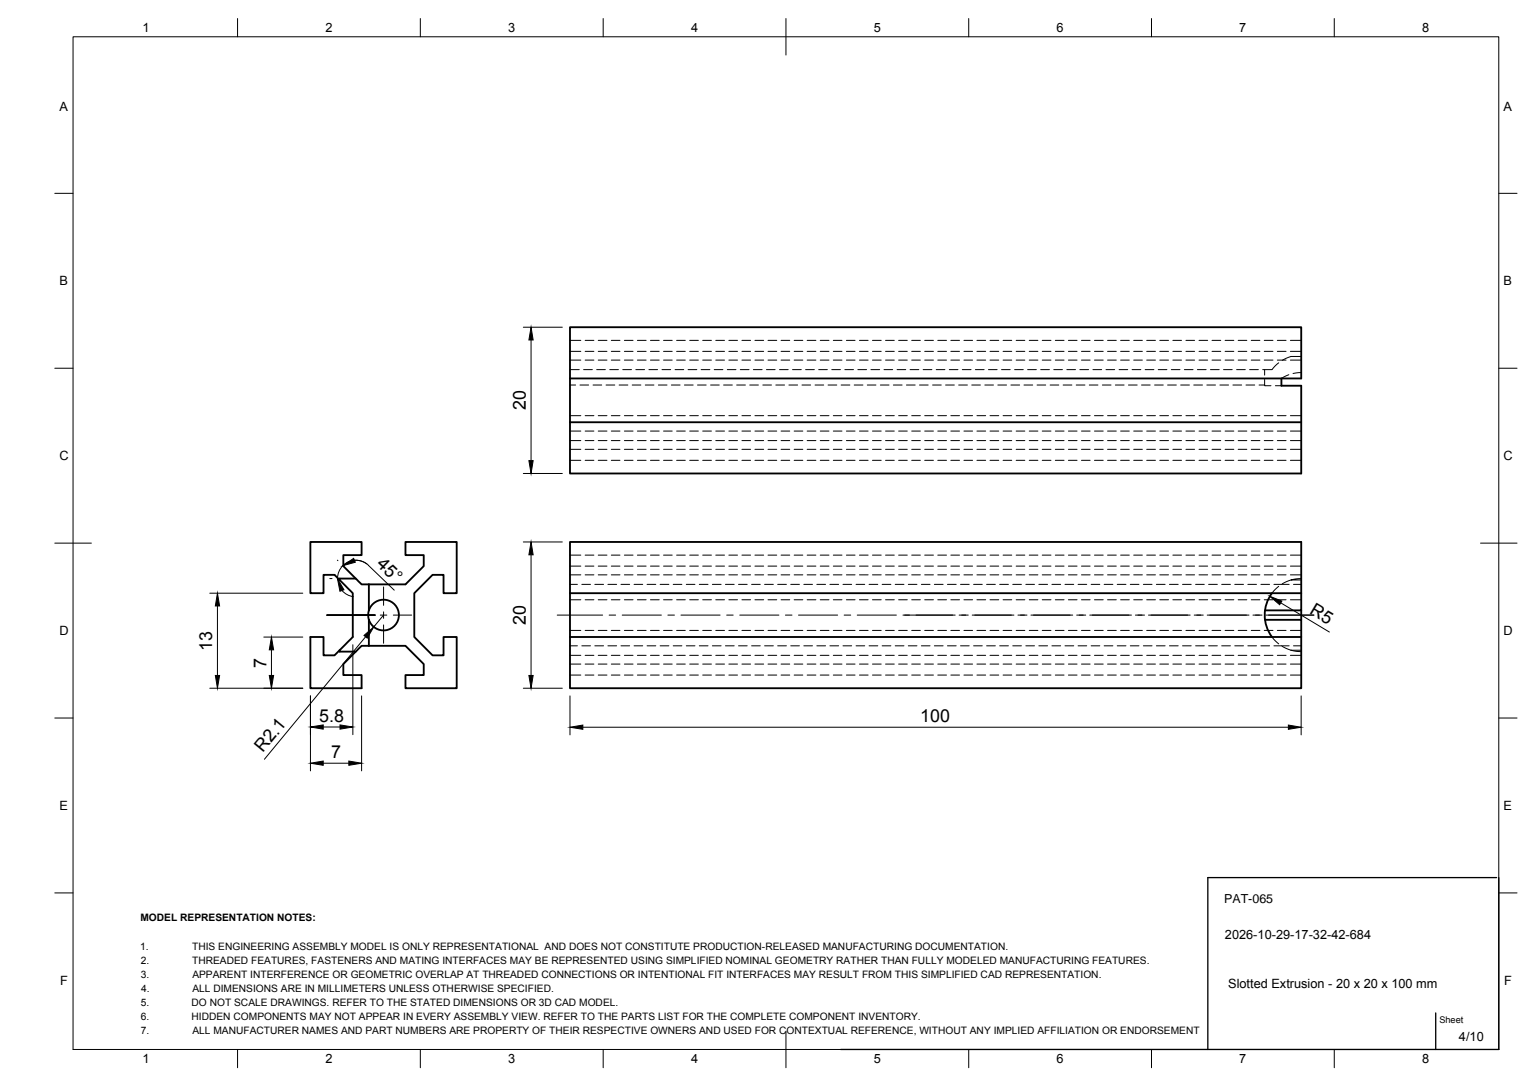
ISO-10303-21;
HEADER;
/* Generated by software containing ST-Developer
 * from STEP Tools, Inc. (www.steptools.com) 
 */

FILE_DESCRIPTION(
/* description */ ('PAT-065'),
/* implementation_level */ '2;1');

FILE_NAME(
/* name */ 'Slotted Extrusion - 20 x 20 x 100 mm.step',
/* time_stamp */ '2026-10-28T22:09:22-07:00',
/* author */ (''),
/* organization */ (''),
/* preprocessor_version */ 'ST-DEVELOPER v20.2',
/* originating_system */ 'Autodesk Translation Framework v15.17.0.0',
/* authorisation */ '');

FILE_SCHEMA (('AUTOMOTIVE_DESIGN { 1 0 10303 214 3 1 1 }'));
ENDSEC;

DATA;
#10=MECHANICAL_DESIGN_GEOMETRIC_PRESENTATION_REPRESENTATION('',(#159),#5502);
#128=B_SPLINE_CURVE_WITH_KNOTS('',3,(#4608,#4609,#4610,#4611,#4612,#4613),
 .UNSPECIFIED.,.F.,.F.,(4,2,4),(0.899292285450093,0.96236755734344,1.02544282923679),
 .UNSPECIFIED.);
#129=ELLIPSE('',#3350,0.707106781186548,0.5);
#130=ELLIPSE('',#3352,0.707106781186547,0.5);
#131=ELLIPSE('',#3354,0.707106781186548,0.5);
#132=ELLIPSE('',#3355,0.707106781186548,0.5);
#139=SHAPE_REPRESENTATION_RELATIONSHIP('SRR','None',#5556,#149);
#149=ADVANCED_BREP_SHAPE_REPRESENTATION('',(#169),#5492);
#159=STYLED_ITEM('',(#5708),#169);
#169=MANIFOLD_SOLID_BREP('Body1',#3206);
#183=FACE_BOUND('',#579,.T.);
#207=PLANE('',#3345);
#208=PLANE('',#3347);
#209=PLANE('',#3357);
#210=PLANE('',#3358);
#211=PLANE('',#3359);
#212=PLANE('',#3360);
#213=PLANE('',#3361);
#214=PLANE('',#3362);
#215=PLANE('',#3363);
#216=PLANE('',#3364);
#217=PLANE('',#3367);
#218=PLANE('',#3368);
#219=PLANE('',#3369);
#220=PLANE('',#3370);
#221=PLANE('',#3371);
#222=PLANE('',#3372);
#223=PLANE('',#3373);
#224=PLANE('',#3374);
#225=PLANE('',#3375);
#226=PLANE('',#3376);
#227=PLANE('',#3377);
#228=PLANE('',#3378);
#229=PLANE('',#3379);
#230=PLANE('',#3380);
#231=PLANE('',#3381);
#232=PLANE('',#3382);
#233=PLANE('',#3383);
#234=PLANE('',#3384);
#235=PLANE('',#3385);
#236=PLANE('',#3386);
#237=PLANE('',#3387);
#238=PLANE('',#3388);
#239=PLANE('',#3389);
#240=PLANE('',#3390);
#241=PLANE('',#3391);
#242=PLANE('',#3392);
#243=PLANE('',#3393);
#244=PLANE('',#3394);
#245=PLANE('',#3395);
#246=PLANE('',#3396);
#247=PLANE('',#3397);
#248=PLANE('',#3398);
#249=PLANE('',#3401);
#250=PLANE('',#3402);
#251=PLANE('',#3403);
#252=PLANE('',#3404);
#253=PLANE('',#3405);
#254=PLANE('',#3406);
#255=PLANE('',#3407);
#256=PLANE('',#3408);
#257=PLANE('',#3409);
#258=PLANE('',#3410);
#346=FACE_OUTER_BOUND('',#526,.T.);
#347=FACE_OUTER_BOUND('',#527,.T.);
#348=FACE_OUTER_BOUND('',#528,.T.);
#349=FACE_OUTER_BOUND('',#529,.T.);
#350=FACE_OUTER_BOUND('',#530,.T.);
#351=FACE_OUTER_BOUND('',#531,.T.);
#352=FACE_OUTER_BOUND('',#532,.T.);
#353=FACE_OUTER_BOUND('',#533,.T.);
#354=FACE_OUTER_BOUND('',#534,.T.);
#355=FACE_OUTER_BOUND('',#535,.T.);
#356=FACE_OUTER_BOUND('',#536,.T.);
#357=FACE_OUTER_BOUND('',#537,.T.);
#358=FACE_OUTER_BOUND('',#538,.T.);
#359=FACE_OUTER_BOUND('',#539,.T.);
#360=FACE_OUTER_BOUND('',#540,.T.);
#361=FACE_OUTER_BOUND('',#541,.T.);
#362=FACE_OUTER_BOUND('',#542,.T.);
#363=FACE_OUTER_BOUND('',#543,.T.);
#364=FACE_OUTER_BOUND('',#544,.T.);
#365=FACE_OUTER_BOUND('',#545,.T.);
#366=FACE_OUTER_BOUND('',#546,.T.);
#367=FACE_OUTER_BOUND('',#547,.T.);
#368=FACE_OUTER_BOUND('',#548,.T.);
#369=FACE_OUTER_BOUND('',#549,.T.);
#370=FACE_OUTER_BOUND('',#550,.T.);
#371=FACE_OUTER_BOUND('',#551,.T.);
#372=FACE_OUTER_BOUND('',#552,.T.);
#373=FACE_OUTER_BOUND('',#553,.T.);
#374=FACE_OUTER_BOUND('',#554,.T.);
#375=FACE_OUTER_BOUND('',#555,.T.);
#376=FACE_OUTER_BOUND('',#556,.T.);
#377=FACE_OUTER_BOUND('',#557,.T.);
#378=FACE_OUTER_BOUND('',#558,.T.);
#379=FACE_OUTER_BOUND('',#559,.T.);
#380=FACE_OUTER_BOUND('',#560,.T.);
#381=FACE_OUTER_BOUND('',#561,.T.);
#382=FACE_OUTER_BOUND('',#562,.T.);
#383=FACE_OUTER_BOUND('',#563,.T.);
#384=FACE_OUTER_BOUND('',#564,.T.);
#385=FACE_OUTER_BOUND('',#565,.T.);
#386=FACE_OUTER_BOUND('',#566,.T.);
#387=FACE_OUTER_BOUND('',#567,.T.);
#388=FACE_OUTER_BOUND('',#568,.T.);
#389=FACE_OUTER_BOUND('',#569,.T.);
#390=FACE_OUTER_BOUND('',#570,.T.);
#391=FACE_OUTER_BOUND('',#571,.T.);
#392=FACE_OUTER_BOUND('',#572,.T.);
#393=FACE_OUTER_BOUND('',#573,.T.);
#394=FACE_OUTER_BOUND('',#574,.T.);
#395=FACE_OUTER_BOUND('',#575,.T.);
#396=FACE_OUTER_BOUND('',#576,.T.);
#397=FACE_OUTER_BOUND('',#577,.T.);
#398=FACE_OUTER_BOUND('',#578,.T.);
#399=FACE_OUTER_BOUND('',#580,.T.);
#526=EDGE_LOOP('',(#2194,#2195,#2196));
#527=EDGE_LOOP('',(#2197,#2198,#2199,#2200));
#528=EDGE_LOOP('',(#2201,#2202,#2203,#2204,#2205,#2206,#2207,#2208,#2209,
#2210,#2211,#2212,#2213,#2214));
#529=EDGE_LOOP('',(#2215,#2216,#2217));
#530=EDGE_LOOP('',(#2218,#2219,#2220,#2221));
#531=EDGE_LOOP('',(#2222,#2223,#2224,#2225));
#532=EDGE_LOOP('',(#2226,#2227,#2228,#2229,#2230,#2231));
#533=EDGE_LOOP('',(#2232,#2233,#2234,#2235,#2236));
#534=EDGE_LOOP('',(#2237,#2238,#2239,#2240,#2241,#2242));
#535=EDGE_LOOP('',(#2243,#2244,#2245,#2246,#2247,#2248,#2249,#2250,#2251,
#2252,#2253,#2254));
#536=EDGE_LOOP('',(#2255,#2256,#2257,#2258,#2259,#2260,#2261,#2262,#2263,
#2264,#2265,#2266,#2267,#2268,#2269,#2270,#2271,#2272,#2273,#2274,#2275,
#2276,#2277,#2278,#2279,#2280,#2281));
#537=EDGE_LOOP('',(#2282,#2283,#2284,#2285));
#538=EDGE_LOOP('',(#2286,#2287,#2288,#2289));
#539=EDGE_LOOP('',(#2290,#2291,#2292,#2293));
#540=EDGE_LOOP('',(#2294,#2295,#2296,#2297,#2298,#2299));
#541=EDGE_LOOP('',(#2300,#2301,#2302,#2303));
#542=EDGE_LOOP('',(#2304,#2305,#2306,#2307));
#543=EDGE_LOOP('',(#2308,#2309,#2310,#2311));
#544=EDGE_LOOP('',(#2312,#2313,#2314,#2315));
#545=EDGE_LOOP('',(#2316,#2317,#2318,#2319));
#546=EDGE_LOOP('',(#2320,#2321,#2322,#2323));
#547=EDGE_LOOP('',(#2324,#2325,#2326,#2327));
#548=EDGE_LOOP('',(#2328,#2329,#2330,#2331,#2332,#2333));
#549=EDGE_LOOP('',(#2334,#2335,#2336,#2337,#2338));
#550=EDGE_LOOP('',(#2339,#2340,#2341,#2342));
#551=EDGE_LOOP('',(#2343,#2344,#2345,#2346));
#552=EDGE_LOOP('',(#2347,#2348,#2349,#2350));
#553=EDGE_LOOP('',(#2351,#2352,#2353,#2354));
#554=EDGE_LOOP('',(#2355,#2356,#2357,#2358));
#555=EDGE_LOOP('',(#2359,#2360,#2361,#2362));
#556=EDGE_LOOP('',(#2363,#2364,#2365,#2366));
#557=EDGE_LOOP('',(#2367,#2368,#2369,#2370));
#558=EDGE_LOOP('',(#2371,#2372,#2373,#2374));
#559=EDGE_LOOP('',(#2375,#2376,#2377,#2378));
#560=EDGE_LOOP('',(#2379,#2380,#2381,#2382));
#561=EDGE_LOOP('',(#2383,#2384,#2385,#2386));
#562=EDGE_LOOP('',(#2387,#2388,#2389,#2390));
#563=EDGE_LOOP('',(#2391,#2392,#2393,#2394));
#564=EDGE_LOOP('',(#2395,#2396,#2397,#2398));
#565=EDGE_LOOP('',(#2399,#2400,#2401,#2402));
#566=EDGE_LOOP('',(#2403,#2404,#2405,#2406));
#567=EDGE_LOOP('',(#2407,#2408,#2409,#2410));
#568=EDGE_LOOP('',(#2411,#2412,#2413,#2414));
#569=EDGE_LOOP('',(#2415,#2416,#2417,#2418,#2419,#2420,#2421,#2422));
#570=EDGE_LOOP('',(#2423,#2424,#2425,#2426));
#571=EDGE_LOOP('',(#2427,#2428,#2429,#2430));
#572=EDGE_LOOP('',(#2431,#2432,#2433,#2434));
#573=EDGE_LOOP('',(#2435,#2436,#2437,#2438));
#574=EDGE_LOOP('',(#2439,#2440,#2441,#2442));
#575=EDGE_LOOP('',(#2443,#2444,#2445,#2446));
#576=EDGE_LOOP('',(#2447,#2448,#2449,#2450));
#577=EDGE_LOOP('',(#2451,#2452,#2453,#2454));
#578=EDGE_LOOP('',(#2455,#2456,#2457,#2458,#2459,#2460,#2461,#2462,#2463,
#2464,#2465,#2466,#2467,#2468,#2469,#2470,#2471,#2472,#2473,#2474,#2475,
#2476,#2477,#2478,#2479,#2480,#2481,#2482,#2483,#2484,#2485,#2486,#2487,
#2488,#2489,#2490,#2491,#2492,#2493,#2494,#2495,#2496,#2497,#2498));
#579=EDGE_LOOP('',(#2499));
#580=EDGE_LOOP('',(#2500,#2501,#2502,#2503,#2504,#2505,#2506,#2507,#2508,
#2509,#2510,#2511));
#724=LINE('',#4581,#1055);
#725=LINE('',#4584,#1056);
#726=LINE('',#4588,#1057);
#727=LINE('',#4592,#1058);
#728=LINE('',#4593,#1059);
#729=LINE('',#4601,#1060);
#730=LINE('',#4605,#1061);
#731=LINE('',#4615,#1062);
#732=LINE('',#4618,#1063);
#733=LINE('',#4624,#1064);
#734=LINE('',#4625,#1065);
#735=LINE('',#4628,#1066);
#736=LINE('',#4630,#1067);
#737=LINE('',#4631,#1068);
#738=LINE('',#4634,#1069);
#739=LINE('',#4636,#1070);
#740=LINE('',#4637,#1071);
#741=LINE('',#4640,#1072);
#742=LINE('',#4642,#1073);
#743=LINE('',#4643,#1074);
#744=LINE('',#4646,#1075);
#745=LINE('',#4648,#1076);
#746=LINE('',#4650,#1077);
#747=LINE('',#4651,#1078);
#748=LINE('',#4654,#1079);
#749=LINE('',#4656,#1080);
#750=LINE('',#4657,#1081);
#751=LINE('',#4660,#1082);
#752=LINE('',#4662,#1083);
#753=LINE('',#4664,#1084);
#754=LINE('',#4666,#1085);
#755=LINE('',#4668,#1086);
#756=LINE('',#4670,#1087);
#757=LINE('',#4672,#1088);
#758=LINE('',#4673,#1089);
#759=LINE('',#4676,#1090);
#760=LINE('',#4678,#1091);
#761=LINE('',#4680,#1092);
#762=LINE('',#4682,#1093);
#763=LINE('',#4684,#1094);
#764=LINE('',#4686,#1095);
#765=LINE('',#4688,#1096);
#766=LINE('',#4690,#1097);
#767=LINE('',#4692,#1098);
#768=LINE('',#4694,#1099);
#769=LINE('',#4696,#1100);
#770=LINE('',#4698,#1101);
#771=LINE('',#4700,#1102);
#772=LINE('',#4702,#1103);
#773=LINE('',#4704,#1104);
#774=LINE('',#4706,#1105);
#775=LINE('',#4708,#1106);
#776=LINE('',#4710,#1107);
#777=LINE('',#4712,#1108);
#778=LINE('',#4714,#1109);
#779=LINE('',#4716,#1110);
#780=LINE('',#4717,#1111);
#781=LINE('',#4724,#1112);
#782=LINE('',#4726,#1113);
#783=LINE('',#4728,#1114);
#784=LINE('',#4729,#1115);
#785=LINE('',#4732,#1116);
#786=LINE('',#4734,#1117);
#787=LINE('',#4735,#1118);
#788=LINE('',#4738,#1119);
#789=LINE('',#4740,#1120);
#790=LINE('',#4741,#1121);
#791=LINE('',#4743,#1122);
#792=LINE('',#4744,#1123);
#793=LINE('',#4747,#1124);
#794=LINE('',#4748,#1125);
#795=LINE('',#4751,#1126);
#796=LINE('',#4752,#1127);
#797=LINE('',#4755,#1128);
#798=LINE('',#4756,#1129);
#799=LINE('',#4759,#1130);
#800=LINE('',#4761,#1131);
#801=LINE('',#4762,#1132);
#802=LINE('',#4765,#1133);
#803=LINE('',#4766,#1134);
#804=LINE('',#4769,#1135);
#805=LINE('',#4770,#1136);
#806=LINE('',#4773,#1137);
#807=LINE('',#4774,#1138);
#808=LINE('',#4777,#1139);
#809=LINE('',#4778,#1140);
#810=LINE('',#4781,#1141);
#811=LINE('',#4783,#1142);
#812=LINE('',#4784,#1143);
#813=LINE('',#4787,#1144);
#814=LINE('',#4789,#1145);
#815=LINE('',#4790,#1146);
#816=LINE('',#4793,#1147);
#817=LINE('',#4795,#1148);
#818=LINE('',#4796,#1149);
#819=LINE('',#4799,#1150);
#820=LINE('',#4801,#1151);
#821=LINE('',#4802,#1152);
#822=LINE('',#4805,#1153);
#823=LINE('',#4807,#1154);
#824=LINE('',#4808,#1155);
#825=LINE('',#4811,#1156);
#826=LINE('',#4812,#1157);
#827=LINE('',#4815,#1158);
#828=LINE('',#4816,#1159);
#829=LINE('',#4819,#1160);
#830=LINE('',#4820,#1161);
#831=LINE('',#4823,#1162);
#832=LINE('',#4824,#1163);
#833=LINE('',#4827,#1164);
#834=LINE('',#4828,#1165);
#835=LINE('',#4831,#1166);
#836=LINE('',#4832,#1167);
#837=LINE('',#4835,#1168);
#838=LINE('',#4836,#1169);
#839=LINE('',#4839,#1170);
#840=LINE('',#4840,#1171);
#841=LINE('',#4843,#1172);
#842=LINE('',#4845,#1173);
#843=LINE('',#4846,#1174);
#844=LINE('',#4849,#1175);
#845=LINE('',#4850,#1176);
#846=LINE('',#4852,#1177);
#847=LINE('',#4855,#1178);
#848=LINE('',#4856,#1179);
#849=LINE('',#4859,#1180);
#850=LINE('',#4860,#1181);
#851=LINE('',#4863,#1182);
#852=LINE('',#4864,#1183);
#853=LINE('',#4867,#1184);
#854=LINE('',#4868,#1185);
#855=LINE('',#4871,#1186);
#856=LINE('',#4875,#1187);
#857=LINE('',#4876,#1188);
#858=LINE('',#4879,#1189);
#859=LINE('',#4881,#1190);
#860=LINE('',#4882,#1191);
#861=LINE('',#4884,#1192);
#862=LINE('',#4885,#1193);
#863=LINE('',#4888,#1194);
#864=LINE('',#4889,#1195);
#865=LINE('',#4891,#1196);
#866=LINE('',#4894,#1197);
#867=LINE('',#4895,#1198);
#868=LINE('',#4897,#1199);
#869=LINE('',#4899,#1200);
#1055=VECTOR('',#3671,1.);
#1056=VECTOR('',#3674,1.);
#1057=VECTOR('',#3677,1.);
#1058=VECTOR('',#3680,1.);
#1059=VECTOR('',#3681,1.);
#1060=VECTOR('',#3688,1.);
#1061=VECTOR('',#3691,1.);
#1062=VECTOR('',#3694,1.);
#1063=VECTOR('',#3697,1.);
#1064=VECTOR('',#3704,1.);
#1065=VECTOR('',#3705,1.);
#1066=VECTOR('',#3708,1.);
#1067=VECTOR('',#3709,1.);
#1068=VECTOR('',#3710,1.);
#1069=VECTOR('',#3713,1.);
#1070=VECTOR('',#3714,1.);
#1071=VECTOR('',#3715,1.);
#1072=VECTOR('',#3718,1.);
#1073=VECTOR('',#3719,1.);
#1074=VECTOR('',#3720,1.);
#1075=VECTOR('',#3723,1.);
#1076=VECTOR('',#3724,1.);
#1077=VECTOR('',#3725,1.);
#1078=VECTOR('',#3726,1.);
#1079=VECTOR('',#3729,1.);
#1080=VECTOR('',#3730,1.);
#1081=VECTOR('',#3731,1.);
#1082=VECTOR('',#3734,1.);
#1083=VECTOR('',#3735,1.);
#1084=VECTOR('',#3736,1.);
#1085=VECTOR('',#3737,1.);
#1086=VECTOR('',#3738,1.);
#1087=VECTOR('',#3739,1.);
#1088=VECTOR('',#3740,1.);
#1089=VECTOR('',#3741,1.);
#1090=VECTOR('',#3744,1.);
#1091=VECTOR('',#3745,1.);
#1092=VECTOR('',#3746,1.);
#1093=VECTOR('',#3747,1.);
#1094=VECTOR('',#3748,1.);
#1095=VECTOR('',#3749,1.);
#1096=VECTOR('',#3750,1.);
#1097=VECTOR('',#3751,1.);
#1098=VECTOR('',#3752,1.);
#1099=VECTOR('',#3753,1.);
#1100=VECTOR('',#3754,1.);
#1101=VECTOR('',#3755,1.);
#1102=VECTOR('',#3756,1.);
#1103=VECTOR('',#3757,1.);
#1104=VECTOR('',#3758,1.);
#1105=VECTOR('',#3759,1.);
#1106=VECTOR('',#3760,1.);
#1107=VECTOR('',#3761,1.);
#1108=VECTOR('',#3762,1.);
#1109=VECTOR('',#3763,1.);
#1110=VECTOR('',#3764,1.);
#1111=VECTOR('',#3765,1.);
#1112=VECTOR('',#3772,1.);
#1113=VECTOR('',#3773,1.);
#1114=VECTOR('',#3774,1.);
#1115=VECTOR('',#3775,1.);
#1116=VECTOR('',#3778,1.);
#1117=VECTOR('',#3779,1.);
#1118=VECTOR('',#3780,1.);
#1119=VECTOR('',#3783,1.);
#1120=VECTOR('',#3784,1.);
#1121=VECTOR('',#3785,1.);
#1122=VECTOR('',#3788,1.);
#1123=VECTOR('',#3789,1.);
#1124=VECTOR('',#3792,1.);
#1125=VECTOR('',#3793,1.);
#1126=VECTOR('',#3796,1.);
#1127=VECTOR('',#3797,1.);
#1128=VECTOR('',#3800,1.);
#1129=VECTOR('',#3801,1.);
#1130=VECTOR('',#3804,1.);
#1131=VECTOR('',#3805,1.);
#1132=VECTOR('',#3806,1.);
#1133=VECTOR('',#3809,1.);
#1134=VECTOR('',#3810,1.);
#1135=VECTOR('',#3813,1.);
#1136=VECTOR('',#3814,1.);
#1137=VECTOR('',#3817,1.);
#1138=VECTOR('',#3818,1.);
#1139=VECTOR('',#3821,1.);
#1140=VECTOR('',#3822,1.);
#1141=VECTOR('',#3825,1.);
#1142=VECTOR('',#3826,1.);
#1143=VECTOR('',#3827,1.);
#1144=VECTOR('',#3830,1.);
#1145=VECTOR('',#3831,1.);
#1146=VECTOR('',#3832,1.);
#1147=VECTOR('',#3835,1.);
#1148=VECTOR('',#3836,1.);
#1149=VECTOR('',#3837,1.);
#1150=VECTOR('',#3840,1.);
#1151=VECTOR('',#3841,1.);
#1152=VECTOR('',#3842,1.);
#1153=VECTOR('',#3845,1.);
#1154=VECTOR('',#3846,1.);
#1155=VECTOR('',#3847,1.);
#1156=VECTOR('',#3850,1.);
#1157=VECTOR('',#3851,1.);
#1158=VECTOR('',#3854,1.);
#1159=VECTOR('',#3855,1.);
#1160=VECTOR('',#3858,1.);
#1161=VECTOR('',#3859,1.);
#1162=VECTOR('',#3862,1.);
#1163=VECTOR('',#3863,1.);
#1164=VECTOR('',#3866,1.);
#1165=VECTOR('',#3867,1.);
#1166=VECTOR('',#3870,1.);
#1167=VECTOR('',#3871,1.);
#1168=VECTOR('',#3874,1.);
#1169=VECTOR('',#3875,1.);
#1170=VECTOR('',#3878,1.);
#1171=VECTOR('',#3879,1.);
#1172=VECTOR('',#3882,1.);
#1173=VECTOR('',#3883,1.);
#1174=VECTOR('',#3884,1.);
#1175=VECTOR('',#3887,1.);
#1176=VECTOR('',#3888,1.);
#1177=VECTOR('',#3891,1.);
#1178=VECTOR('',#3894,1.);
#1179=VECTOR('',#3895,1.);
#1180=VECTOR('',#3898,1.);
#1181=VECTOR('',#3899,1.);
#1182=VECTOR('',#3902,1.);
#1183=VECTOR('',#3903,1.);
#1184=VECTOR('',#3906,1.);
#1185=VECTOR('',#3907,1.);
#1186=VECTOR('',#3910,0.21);
#1187=VECTOR('',#3915,1.);
#1188=VECTOR('',#3916,1.);
#1189=VECTOR('',#3919,1.);
#1190=VECTOR('',#3920,1.);
#1191=VECTOR('',#3921,1.);
#1192=VECTOR('',#3924,1.);
#1193=VECTOR('',#3925,1.);
#1194=VECTOR('',#3928,1.);
#1195=VECTOR('',#3929,1.);
#1196=VECTOR('',#3932,1.);
#1197=VECTOR('',#3935,1.);
#1198=VECTOR('',#3936,1.);
#1199=VECTOR('',#3939,1.);
#1200=VECTOR('',#3942,1.);
#1377=CIRCLE('',#3346,0.5);
#1378=CIRCLE('',#3348,0.5);
#1379=CIRCLE('',#3351,0.5);
#1380=CIRCLE('',#3353,0.5);
#1381=CIRCLE('',#3356,0.5);
#1382=CIRCLE('',#3365,0.21);
#1383=CIRCLE('',#3366,0.21);
#1384=CIRCLE('',#3400,0.21);
#1458=VERTEX_POINT('',#4579);
#1459=VERTEX_POINT('',#4580);
#1460=VERTEX_POINT('',#4582);
#1461=VERTEX_POINT('',#4586);
#1462=VERTEX_POINT('',#4587);
#1463=VERTEX_POINT('',#4589);
#1464=VERTEX_POINT('',#4591);
#1465=VERTEX_POINT('',#4595);
#1466=VERTEX_POINT('',#4596);
#1467=VERTEX_POINT('',#4598);
#1468=VERTEX_POINT('',#4600);
#1469=VERTEX_POINT('',#4602);
#1470=VERTEX_POINT('',#4604);
#1471=VERTEX_POINT('',#4606);
#1472=VERTEX_POINT('',#4614);
#1473=VERTEX_POINT('',#4616);
#1474=VERTEX_POINT('',#4619);
#1475=VERTEX_POINT('',#4623);
#1476=VERTEX_POINT('',#4627);
#1477=VERTEX_POINT('',#4629);
#1478=VERTEX_POINT('',#4633);
#1479=VERTEX_POINT('',#4635);
#1480=VERTEX_POINT('',#4639);
#1481=VERTEX_POINT('',#4641);
#1482=VERTEX_POINT('',#4645);
#1483=VERTEX_POINT('',#4647);
#1484=VERTEX_POINT('',#4649);
#1485=VERTEX_POINT('',#4653);
#1486=VERTEX_POINT('',#4655);
#1487=VERTEX_POINT('',#4659);
#1488=VERTEX_POINT('',#4661);
#1489=VERTEX_POINT('',#4663);
#1490=VERTEX_POINT('',#4665);
#1491=VERTEX_POINT('',#4667);
#1492=VERTEX_POINT('',#4669);
#1493=VERTEX_POINT('',#4671);
#1494=VERTEX_POINT('',#4675);
#1495=VERTEX_POINT('',#4677);
#1496=VERTEX_POINT('',#4679);
#1497=VERTEX_POINT('',#4681);
#1498=VERTEX_POINT('',#4683);
#1499=VERTEX_POINT('',#4685);
#1500=VERTEX_POINT('',#4687);
#1501=VERTEX_POINT('',#4689);
#1502=VERTEX_POINT('',#4691);
#1503=VERTEX_POINT('',#4693);
#1504=VERTEX_POINT('',#4695);
#1505=VERTEX_POINT('',#4697);
#1506=VERTEX_POINT('',#4699);
#1507=VERTEX_POINT('',#4701);
#1508=VERTEX_POINT('',#4703);
#1509=VERTEX_POINT('',#4705);
#1510=VERTEX_POINT('',#4707);
#1511=VERTEX_POINT('',#4709);
#1512=VERTEX_POINT('',#4711);
#1513=VERTEX_POINT('',#4713);
#1514=VERTEX_POINT('',#4715);
#1515=VERTEX_POINT('',#4718);
#1516=VERTEX_POINT('',#4722);
#1517=VERTEX_POINT('',#4723);
#1518=VERTEX_POINT('',#4725);
#1519=VERTEX_POINT('',#4727);
#1520=VERTEX_POINT('',#4731);
#1521=VERTEX_POINT('',#4733);
#1522=VERTEX_POINT('',#4737);
#1523=VERTEX_POINT('',#4739);
#1524=VERTEX_POINT('',#4746);
#1525=VERTEX_POINT('',#4750);
#1526=VERTEX_POINT('',#4754);
#1527=VERTEX_POINT('',#4758);
#1528=VERTEX_POINT('',#4760);
#1529=VERTEX_POINT('',#4764);
#1530=VERTEX_POINT('',#4768);
#1531=VERTEX_POINT('',#4772);
#1532=VERTEX_POINT('',#4776);
#1533=VERTEX_POINT('',#4780);
#1534=VERTEX_POINT('',#4782);
#1535=VERTEX_POINT('',#4786);
#1536=VERTEX_POINT('',#4788);
#1537=VERTEX_POINT('',#4792);
#1538=VERTEX_POINT('',#4794);
#1539=VERTEX_POINT('',#4798);
#1540=VERTEX_POINT('',#4800);
#1541=VERTEX_POINT('',#4804);
#1542=VERTEX_POINT('',#4806);
#1543=VERTEX_POINT('',#4810);
#1544=VERTEX_POINT('',#4814);
#1545=VERTEX_POINT('',#4818);
#1546=VERTEX_POINT('',#4822);
#1547=VERTEX_POINT('',#4826);
#1548=VERTEX_POINT('',#4830);
#1549=VERTEX_POINT('',#4834);
#1550=VERTEX_POINT('',#4838);
#1551=VERTEX_POINT('',#4842);
#1552=VERTEX_POINT('',#4844);
#1553=VERTEX_POINT('',#4848);
#1554=VERTEX_POINT('',#4854);
#1555=VERTEX_POINT('',#4858);
#1556=VERTEX_POINT('',#4862);
#1557=VERTEX_POINT('',#4866);
#1558=VERTEX_POINT('',#4870);
#1559=VERTEX_POINT('',#4874);
#1560=VERTEX_POINT('',#4878);
#1561=VERTEX_POINT('',#4880);
#1562=VERTEX_POINT('',#4887);
#1563=VERTEX_POINT('',#4893);
#1747=EDGE_CURVE('',#1458,#1459,#724,.T.);
#1748=EDGE_CURVE('',#1460,#1458,#1377,.T.);
#1749=EDGE_CURVE('',#1459,#1460,#725,.T.);
#1750=EDGE_CURVE('',#1461,#1462,#726,.T.);
#1751=EDGE_CURVE('',#1461,#1463,#1378,.T.);
#1752=EDGE_CURVE('',#1464,#1463,#727,.T.);
#1753=EDGE_CURVE('',#1462,#1464,#728,.T.);
#1754=EDGE_CURVE('',#1465,#1466,#129,.T.);
#1755=EDGE_CURVE('',#1465,#1467,#1379,.T.);
#1756=EDGE_CURVE('',#1468,#1467,#729,.T.);
#1757=EDGE_CURVE('',#1469,#1468,#130,.T.);
#1758=EDGE_CURVE('',#1470,#1469,#730,.T.);
#1759=EDGE_CURVE('',#1471,#1470,#1380,.T.);
#1760=EDGE_CURVE('',#1463,#1471,#128,.T.);
#1761=EDGE_CURVE('',#1472,#1461,#731,.T.);
#1762=EDGE_CURVE('',#1473,#1472,#131,.T.);
#1763=EDGE_CURVE('',#1460,#1473,#732,.T.);
#1764=EDGE_CURVE('',#1474,#1458,#132,.T.);
#1765=EDGE_CURVE('',#1466,#1474,#1381,.T.);
#1766=EDGE_CURVE('',#1475,#1465,#733,.T.);
#1767=EDGE_CURVE('',#1467,#1475,#734,.T.);
#1768=EDGE_CURVE('',#1476,#1470,#735,.T.);
#1769=EDGE_CURVE('',#1477,#1476,#736,.T.);
#1770=EDGE_CURVE('',#1471,#1477,#737,.T.);
#1771=EDGE_CURVE('',#1474,#1478,#738,.T.);
#1772=EDGE_CURVE('',#1479,#1478,#739,.T.);
#1773=EDGE_CURVE('',#1466,#1479,#740,.T.);
#1774=EDGE_CURVE('',#1480,#1459,#741,.T.);
#1775=EDGE_CURVE('',#1480,#1481,#742,.T.);
#1776=EDGE_CURVE('',#1478,#1481,#743,.T.);
#1777=EDGE_CURVE('',#1472,#1482,#744,.T.);
#1778=EDGE_CURVE('',#1483,#1482,#745,.T.);
#1779=EDGE_CURVE('',#1484,#1483,#746,.T.);
#1780=EDGE_CURVE('',#1473,#1484,#747,.T.);
#1781=EDGE_CURVE('',#1485,#1462,#748,.T.);
#1782=EDGE_CURVE('',#1485,#1486,#749,.T.);
#1783=EDGE_CURVE('',#1482,#1486,#750,.T.);
#1784=EDGE_CURVE('',#1484,#1487,#751,.T.);
#1785=EDGE_CURVE('',#1487,#1488,#752,.T.);
#1786=EDGE_CURVE('',#1488,#1489,#753,.T.);
#1787=EDGE_CURVE('',#1490,#1489,#754,.T.);
#1788=EDGE_CURVE('',#1491,#1490,#755,.T.);
#1789=EDGE_CURVE('',#1491,#1492,#756,.T.);
#1790=EDGE_CURVE('',#1492,#1493,#757,.T.);
#1791=EDGE_CURVE('',#1493,#1480,#758,.T.);
#1792=EDGE_CURVE('',#1476,#1494,#759,.T.);
#1793=EDGE_CURVE('',#1494,#1495,#760,.T.);
#1794=EDGE_CURVE('',#1495,#1496,#761,.T.);
#1795=EDGE_CURVE('',#1496,#1497,#762,.T.);
#1796=EDGE_CURVE('',#1497,#1498,#763,.T.);
#1797=EDGE_CURVE('',#1499,#1498,#764,.T.);
#1798=EDGE_CURVE('',#1500,#1499,#765,.T.);
#1799=EDGE_CURVE('',#1500,#1501,#766,.T.);
#1800=EDGE_CURVE('',#1501,#1502,#767,.T.);
#1801=EDGE_CURVE('',#1502,#1503,#768,.T.);
#1802=EDGE_CURVE('',#1503,#1504,#769,.T.);
#1803=EDGE_CURVE('',#1504,#1505,#770,.T.);
#1804=EDGE_CURVE('',#1505,#1506,#771,.T.);
#1805=EDGE_CURVE('',#1506,#1507,#772,.T.);
#1806=EDGE_CURVE('',#1507,#1508,#773,.T.);
#1807=EDGE_CURVE('',#1508,#1509,#774,.T.);
#1808=EDGE_CURVE('',#1510,#1509,#775,.T.);
#1809=EDGE_CURVE('',#1511,#1510,#776,.T.);
#1810=EDGE_CURVE('',#1511,#1512,#777,.T.);
#1811=EDGE_CURVE('',#1512,#1513,#778,.T.);
#1812=EDGE_CURVE('',#1513,#1514,#779,.T.);
#1813=EDGE_CURVE('',#1514,#1485,#780,.T.);
#1814=EDGE_CURVE('',#1464,#1515,#1382,.T.);
#1815=EDGE_CURVE('',#1515,#1477,#1383,.T.);
#1816=EDGE_CURVE('',#1516,#1517,#781,.T.);
#1817=EDGE_CURVE('',#1516,#1518,#782,.T.);
#1818=EDGE_CURVE('',#1519,#1518,#783,.T.);
#1819=EDGE_CURVE('',#1517,#1519,#784,.T.);
#1820=EDGE_CURVE('',#1520,#1516,#785,.T.);
#1821=EDGE_CURVE('',#1520,#1521,#786,.T.);
#1822=EDGE_CURVE('',#1518,#1521,#787,.T.);
#1823=EDGE_CURVE('',#1522,#1520,#788,.T.);
#1824=EDGE_CURVE('',#1522,#1523,#789,.T.);
#1825=EDGE_CURVE('',#1521,#1523,#790,.T.);
#1826=EDGE_CURVE('',#1523,#1479,#791,.T.);
#1827=EDGE_CURVE('',#1475,#1522,#792,.T.);
#1828=EDGE_CURVE('',#1493,#1524,#793,.T.);
#1829=EDGE_CURVE('',#1481,#1524,#794,.T.);
#1830=EDGE_CURVE('',#1492,#1525,#795,.T.);
#1831=EDGE_CURVE('',#1524,#1525,#796,.T.);
#1832=EDGE_CURVE('',#1526,#1491,#797,.T.);
#1833=EDGE_CURVE('',#1525,#1526,#798,.T.);
#1834=EDGE_CURVE('',#1497,#1527,#799,.T.);
#1835=EDGE_CURVE('',#1528,#1527,#800,.T.);
#1836=EDGE_CURVE('',#1498,#1528,#801,.T.);
#1837=EDGE_CURVE('',#1496,#1529,#802,.T.);
#1838=EDGE_CURVE('',#1527,#1529,#803,.T.);
#1839=EDGE_CURVE('',#1495,#1530,#804,.T.);
#1840=EDGE_CURVE('',#1529,#1530,#805,.T.);
#1841=EDGE_CURVE('',#1494,#1531,#806,.T.);
#1842=EDGE_CURVE('',#1530,#1531,#807,.T.);
#1843=EDGE_CURVE('',#1469,#1532,#808,.T.);
#1844=EDGE_CURVE('',#1531,#1532,#809,.T.);
#1845=EDGE_CURVE('',#1533,#1468,#810,.T.);
#1846=EDGE_CURVE('',#1533,#1534,#811,.T.);
#1847=EDGE_CURVE('',#1532,#1534,#812,.T.);
#1848=EDGE_CURVE('',#1535,#1533,#813,.T.);
#1849=EDGE_CURVE('',#1535,#1536,#814,.T.);
#1850=EDGE_CURVE('',#1534,#1536,#815,.T.);
#1851=EDGE_CURVE('',#1537,#1535,#816,.T.);
#1852=EDGE_CURVE('',#1537,#1538,#817,.T.);
#1853=EDGE_CURVE('',#1536,#1538,#818,.T.);
#1854=EDGE_CURVE('',#1539,#1537,#819,.T.);
#1855=EDGE_CURVE('',#1540,#1539,#820,.T.);
#1856=EDGE_CURVE('',#1538,#1540,#821,.T.);
#1857=EDGE_CURVE('',#1508,#1541,#822,.T.);
#1858=EDGE_CURVE('',#1542,#1541,#823,.T.);
#1859=EDGE_CURVE('',#1509,#1542,#824,.T.);
#1860=EDGE_CURVE('',#1507,#1543,#825,.T.);
#1861=EDGE_CURVE('',#1541,#1543,#826,.T.);
#1862=EDGE_CURVE('',#1506,#1544,#827,.T.);
#1863=EDGE_CURVE('',#1543,#1544,#828,.T.);
#1864=EDGE_CURVE('',#1505,#1545,#829,.T.);
#1865=EDGE_CURVE('',#1544,#1545,#830,.T.);
#1866=EDGE_CURVE('',#1504,#1546,#831,.T.);
#1867=EDGE_CURVE('',#1545,#1546,#832,.T.);
#1868=EDGE_CURVE('',#1503,#1547,#833,.T.);
#1869=EDGE_CURVE('',#1546,#1547,#834,.T.);
#1870=EDGE_CURVE('',#1502,#1548,#835,.T.);
#1871=EDGE_CURVE('',#1547,#1548,#836,.T.);
#1872=EDGE_CURVE('',#1501,#1549,#837,.T.);
#1873=EDGE_CURVE('',#1548,#1549,#838,.T.);
#1874=EDGE_CURVE('',#1550,#1500,#839,.T.);
#1875=EDGE_CURVE('',#1549,#1550,#840,.T.);
#1876=EDGE_CURVE('',#1488,#1551,#841,.T.);
#1877=EDGE_CURVE('',#1552,#1551,#842,.T.);
#1878=EDGE_CURVE('',#1489,#1552,#843,.T.);
#1879=EDGE_CURVE('',#1487,#1553,#844,.T.);
#1880=EDGE_CURVE('',#1551,#1553,#845,.T.);
#1881=EDGE_CURVE('',#1553,#1483,#846,.T.);
#1882=EDGE_CURVE('',#1514,#1554,#847,.T.);
#1883=EDGE_CURVE('',#1486,#1554,#848,.T.);
#1884=EDGE_CURVE('',#1513,#1555,#849,.T.);
#1885=EDGE_CURVE('',#1554,#1555,#850,.T.);
#1886=EDGE_CURVE('',#1512,#1556,#851,.T.);
#1887=EDGE_CURVE('',#1555,#1556,#852,.T.);
#1888=EDGE_CURVE('',#1557,#1511,#853,.T.);
#1889=EDGE_CURVE('',#1556,#1557,#854,.T.);
#1890=EDGE_CURVE('',#1515,#1558,#855,.T.);
#1891=EDGE_CURVE('',#1558,#1558,#1384,.T.);
#1892=EDGE_CURVE('',#1490,#1559,#856,.T.);
#1893=EDGE_CURVE('',#1526,#1559,#857,.T.);
#1894=EDGE_CURVE('',#1560,#1519,#858,.T.);
#1895=EDGE_CURVE('',#1561,#1560,#859,.T.);
#1896=EDGE_CURVE('',#1561,#1517,#860,.T.);
#1897=EDGE_CURVE('',#1539,#1561,#861,.T.);
#1898=EDGE_CURVE('',#1540,#1560,#862,.T.);
#1899=EDGE_CURVE('',#1562,#1528,#863,.T.);
#1900=EDGE_CURVE('',#1499,#1562,#864,.T.);
#1901=EDGE_CURVE('',#1550,#1562,#865,.T.);
#1902=EDGE_CURVE('',#1563,#1542,#866,.T.);
#1903=EDGE_CURVE('',#1510,#1563,#867,.T.);
#1904=EDGE_CURVE('',#1557,#1563,#868,.T.);
#1905=EDGE_CURVE('',#1559,#1552,#869,.T.);
#2194=ORIENTED_EDGE('',*,*,#1747,.F.);
#2195=ORIENTED_EDGE('',*,*,#1748,.F.);
#2196=ORIENTED_EDGE('',*,*,#1749,.F.);
#2197=ORIENTED_EDGE('',*,*,#1750,.F.);
#2198=ORIENTED_EDGE('',*,*,#1751,.T.);
#2199=ORIENTED_EDGE('',*,*,#1752,.F.);
#2200=ORIENTED_EDGE('',*,*,#1753,.F.);
#2201=ORIENTED_EDGE('',*,*,#1754,.F.);
#2202=ORIENTED_EDGE('',*,*,#1755,.T.);
#2203=ORIENTED_EDGE('',*,*,#1756,.F.);
#2204=ORIENTED_EDGE('',*,*,#1757,.F.);
#2205=ORIENTED_EDGE('',*,*,#1758,.F.);
#2206=ORIENTED_EDGE('',*,*,#1759,.F.);
#2207=ORIENTED_EDGE('',*,*,#1760,.F.);
#2208=ORIENTED_EDGE('',*,*,#1751,.F.);
#2209=ORIENTED_EDGE('',*,*,#1761,.F.);
#2210=ORIENTED_EDGE('',*,*,#1762,.F.);
#2211=ORIENTED_EDGE('',*,*,#1763,.F.);
#2212=ORIENTED_EDGE('',*,*,#1748,.T.);
#2213=ORIENTED_EDGE('',*,*,#1764,.F.);
#2214=ORIENTED_EDGE('',*,*,#1765,.F.);
#2215=ORIENTED_EDGE('',*,*,#1766,.F.);
#2216=ORIENTED_EDGE('',*,*,#1767,.F.);
#2217=ORIENTED_EDGE('',*,*,#1755,.F.);
#2218=ORIENTED_EDGE('',*,*,#1768,.F.);
#2219=ORIENTED_EDGE('',*,*,#1769,.F.);
#2220=ORIENTED_EDGE('',*,*,#1770,.F.);
#2221=ORIENTED_EDGE('',*,*,#1759,.T.);
#2222=ORIENTED_EDGE('',*,*,#1765,.T.);
#2223=ORIENTED_EDGE('',*,*,#1771,.T.);
#2224=ORIENTED_EDGE('',*,*,#1772,.F.);
#2225=ORIENTED_EDGE('',*,*,#1773,.F.);
#2226=ORIENTED_EDGE('',*,*,#1764,.T.);
#2227=ORIENTED_EDGE('',*,*,#1747,.T.);
#2228=ORIENTED_EDGE('',*,*,#1774,.F.);
#2229=ORIENTED_EDGE('',*,*,#1775,.T.);
#2230=ORIENTED_EDGE('',*,*,#1776,.F.);
#2231=ORIENTED_EDGE('',*,*,#1771,.F.);
#2232=ORIENTED_EDGE('',*,*,#1762,.T.);
#2233=ORIENTED_EDGE('',*,*,#1777,.T.);
#2234=ORIENTED_EDGE('',*,*,#1778,.F.);
#2235=ORIENTED_EDGE('',*,*,#1779,.F.);
#2236=ORIENTED_EDGE('',*,*,#1780,.F.);
#2237=ORIENTED_EDGE('',*,*,#1761,.T.);
#2238=ORIENTED_EDGE('',*,*,#1750,.T.);
#2239=ORIENTED_EDGE('',*,*,#1781,.F.);
#2240=ORIENTED_EDGE('',*,*,#1782,.T.);
#2241=ORIENTED_EDGE('',*,*,#1783,.F.);
#2242=ORIENTED_EDGE('',*,*,#1777,.F.);
#2243=ORIENTED_EDGE('',*,*,#1749,.T.);
#2244=ORIENTED_EDGE('',*,*,#1763,.T.);
#2245=ORIENTED_EDGE('',*,*,#1780,.T.);
#2246=ORIENTED_EDGE('',*,*,#1784,.T.);
#2247=ORIENTED_EDGE('',*,*,#1785,.T.);
#2248=ORIENTED_EDGE('',*,*,#1786,.T.);
#2249=ORIENTED_EDGE('',*,*,#1787,.F.);
#2250=ORIENTED_EDGE('',*,*,#1788,.F.);
#2251=ORIENTED_EDGE('',*,*,#1789,.T.);
#2252=ORIENTED_EDGE('',*,*,#1790,.T.);
#2253=ORIENTED_EDGE('',*,*,#1791,.T.);
#2254=ORIENTED_EDGE('',*,*,#1774,.T.);
#2255=ORIENTED_EDGE('',*,*,#1769,.T.);
#2256=ORIENTED_EDGE('',*,*,#1792,.T.);
#2257=ORIENTED_EDGE('',*,*,#1793,.T.);
#2258=ORIENTED_EDGE('',*,*,#1794,.T.);
#2259=ORIENTED_EDGE('',*,*,#1795,.T.);
#2260=ORIENTED_EDGE('',*,*,#1796,.T.);
#2261=ORIENTED_EDGE('',*,*,#1797,.F.);
#2262=ORIENTED_EDGE('',*,*,#1798,.F.);
#2263=ORIENTED_EDGE('',*,*,#1799,.T.);
#2264=ORIENTED_EDGE('',*,*,#1800,.T.);
#2265=ORIENTED_EDGE('',*,*,#1801,.T.);
#2266=ORIENTED_EDGE('',*,*,#1802,.T.);
#2267=ORIENTED_EDGE('',*,*,#1803,.T.);
#2268=ORIENTED_EDGE('',*,*,#1804,.T.);
#2269=ORIENTED_EDGE('',*,*,#1805,.T.);
#2270=ORIENTED_EDGE('',*,*,#1806,.T.);
#2271=ORIENTED_EDGE('',*,*,#1807,.T.);
#2272=ORIENTED_EDGE('',*,*,#1808,.F.);
#2273=ORIENTED_EDGE('',*,*,#1809,.F.);
#2274=ORIENTED_EDGE('',*,*,#1810,.T.);
#2275=ORIENTED_EDGE('',*,*,#1811,.T.);
#2276=ORIENTED_EDGE('',*,*,#1812,.T.);
#2277=ORIENTED_EDGE('',*,*,#1813,.T.);
#2278=ORIENTED_EDGE('',*,*,#1781,.T.);
#2279=ORIENTED_EDGE('',*,*,#1753,.T.);
#2280=ORIENTED_EDGE('',*,*,#1814,.T.);
#2281=ORIENTED_EDGE('',*,*,#1815,.T.);
#2282=ORIENTED_EDGE('',*,*,#1816,.F.);
#2283=ORIENTED_EDGE('',*,*,#1817,.T.);
#2284=ORIENTED_EDGE('',*,*,#1818,.F.);
#2285=ORIENTED_EDGE('',*,*,#1819,.F.);
#2286=ORIENTED_EDGE('',*,*,#1820,.F.);
#2287=ORIENTED_EDGE('',*,*,#1821,.T.);
#2288=ORIENTED_EDGE('',*,*,#1822,.F.);
#2289=ORIENTED_EDGE('',*,*,#1817,.F.);
#2290=ORIENTED_EDGE('',*,*,#1823,.F.);
#2291=ORIENTED_EDGE('',*,*,#1824,.T.);
#2292=ORIENTED_EDGE('',*,*,#1825,.F.);
#2293=ORIENTED_EDGE('',*,*,#1821,.F.);
#2294=ORIENTED_EDGE('',*,*,#1754,.T.);
#2295=ORIENTED_EDGE('',*,*,#1773,.T.);
#2296=ORIENTED_EDGE('',*,*,#1826,.F.);
#2297=ORIENTED_EDGE('',*,*,#1824,.F.);
#2298=ORIENTED_EDGE('',*,*,#1827,.F.);
#2299=ORIENTED_EDGE('',*,*,#1766,.T.);
#2300=ORIENTED_EDGE('',*,*,#1791,.F.);
#2301=ORIENTED_EDGE('',*,*,#1828,.T.);
#2302=ORIENTED_EDGE('',*,*,#1829,.F.);
#2303=ORIENTED_EDGE('',*,*,#1775,.F.);
#2304=ORIENTED_EDGE('',*,*,#1790,.F.);
#2305=ORIENTED_EDGE('',*,*,#1830,.T.);
#2306=ORIENTED_EDGE('',*,*,#1831,.F.);
#2307=ORIENTED_EDGE('',*,*,#1828,.F.);
#2308=ORIENTED_EDGE('',*,*,#1789,.F.);
#2309=ORIENTED_EDGE('',*,*,#1832,.F.);
#2310=ORIENTED_EDGE('',*,*,#1833,.F.);
#2311=ORIENTED_EDGE('',*,*,#1830,.F.);
#2312=ORIENTED_EDGE('',*,*,#1796,.F.);
#2313=ORIENTED_EDGE('',*,*,#1834,.T.);
#2314=ORIENTED_EDGE('',*,*,#1835,.F.);
#2315=ORIENTED_EDGE('',*,*,#1836,.F.);
#2316=ORIENTED_EDGE('',*,*,#1795,.F.);
#2317=ORIENTED_EDGE('',*,*,#1837,.T.);
#2318=ORIENTED_EDGE('',*,*,#1838,.F.);
#2319=ORIENTED_EDGE('',*,*,#1834,.F.);
#2320=ORIENTED_EDGE('',*,*,#1794,.F.);
#2321=ORIENTED_EDGE('',*,*,#1839,.T.);
#2322=ORIENTED_EDGE('',*,*,#1840,.F.);
#2323=ORIENTED_EDGE('',*,*,#1837,.F.);
#2324=ORIENTED_EDGE('',*,*,#1793,.F.);
#2325=ORIENTED_EDGE('',*,*,#1841,.T.);
#2326=ORIENTED_EDGE('',*,*,#1842,.F.);
#2327=ORIENTED_EDGE('',*,*,#1839,.F.);
#2328=ORIENTED_EDGE('',*,*,#1758,.T.);
#2329=ORIENTED_EDGE('',*,*,#1843,.T.);
#2330=ORIENTED_EDGE('',*,*,#1844,.F.);
#2331=ORIENTED_EDGE('',*,*,#1841,.F.);
#2332=ORIENTED_EDGE('',*,*,#1792,.F.);
#2333=ORIENTED_EDGE('',*,*,#1768,.T.);
#2334=ORIENTED_EDGE('',*,*,#1757,.T.);
#2335=ORIENTED_EDGE('',*,*,#1845,.F.);
#2336=ORIENTED_EDGE('',*,*,#1846,.T.);
#2337=ORIENTED_EDGE('',*,*,#1847,.F.);
#2338=ORIENTED_EDGE('',*,*,#1843,.F.);
#2339=ORIENTED_EDGE('',*,*,#1848,.F.);
#2340=ORIENTED_EDGE('',*,*,#1849,.T.);
#2341=ORIENTED_EDGE('',*,*,#1850,.F.);
#2342=ORIENTED_EDGE('',*,*,#1846,.F.);
#2343=ORIENTED_EDGE('',*,*,#1851,.F.);
#2344=ORIENTED_EDGE('',*,*,#1852,.T.);
#2345=ORIENTED_EDGE('',*,*,#1853,.F.);
#2346=ORIENTED_EDGE('',*,*,#1849,.F.);
#2347=ORIENTED_EDGE('',*,*,#1854,.F.);
#2348=ORIENTED_EDGE('',*,*,#1855,.F.);
#2349=ORIENTED_EDGE('',*,*,#1856,.F.);
#2350=ORIENTED_EDGE('',*,*,#1852,.F.);
#2351=ORIENTED_EDGE('',*,*,#1807,.F.);
#2352=ORIENTED_EDGE('',*,*,#1857,.T.);
#2353=ORIENTED_EDGE('',*,*,#1858,.F.);
#2354=ORIENTED_EDGE('',*,*,#1859,.F.);
#2355=ORIENTED_EDGE('',*,*,#1806,.F.);
#2356=ORIENTED_EDGE('',*,*,#1860,.T.);
#2357=ORIENTED_EDGE('',*,*,#1861,.F.);
#2358=ORIENTED_EDGE('',*,*,#1857,.F.);
#2359=ORIENTED_EDGE('',*,*,#1805,.F.);
#2360=ORIENTED_EDGE('',*,*,#1862,.T.);
#2361=ORIENTED_EDGE('',*,*,#1863,.F.);
#2362=ORIENTED_EDGE('',*,*,#1860,.F.);
#2363=ORIENTED_EDGE('',*,*,#1804,.F.);
#2364=ORIENTED_EDGE('',*,*,#1864,.T.);
#2365=ORIENTED_EDGE('',*,*,#1865,.F.);
#2366=ORIENTED_EDGE('',*,*,#1862,.F.);
#2367=ORIENTED_EDGE('',*,*,#1803,.F.);
#2368=ORIENTED_EDGE('',*,*,#1866,.T.);
#2369=ORIENTED_EDGE('',*,*,#1867,.F.);
#2370=ORIENTED_EDGE('',*,*,#1864,.F.);
#2371=ORIENTED_EDGE('',*,*,#1802,.F.);
#2372=ORIENTED_EDGE('',*,*,#1868,.T.);
#2373=ORIENTED_EDGE('',*,*,#1869,.F.);
#2374=ORIENTED_EDGE('',*,*,#1866,.F.);
#2375=ORIENTED_EDGE('',*,*,#1801,.F.);
#2376=ORIENTED_EDGE('',*,*,#1870,.T.);
#2377=ORIENTED_EDGE('',*,*,#1871,.F.);
#2378=ORIENTED_EDGE('',*,*,#1868,.F.);
#2379=ORIENTED_EDGE('',*,*,#1800,.F.);
#2380=ORIENTED_EDGE('',*,*,#1872,.T.);
#2381=ORIENTED_EDGE('',*,*,#1873,.F.);
#2382=ORIENTED_EDGE('',*,*,#1870,.F.);
#2383=ORIENTED_EDGE('',*,*,#1799,.F.);
#2384=ORIENTED_EDGE('',*,*,#1874,.F.);
#2385=ORIENTED_EDGE('',*,*,#1875,.F.);
#2386=ORIENTED_EDGE('',*,*,#1872,.F.);
#2387=ORIENTED_EDGE('',*,*,#1786,.F.);
#2388=ORIENTED_EDGE('',*,*,#1876,.T.);
#2389=ORIENTED_EDGE('',*,*,#1877,.F.);
#2390=ORIENTED_EDGE('',*,*,#1878,.F.);
#2391=ORIENTED_EDGE('',*,*,#1785,.F.);
#2392=ORIENTED_EDGE('',*,*,#1879,.T.);
#2393=ORIENTED_EDGE('',*,*,#1880,.F.);
#2394=ORIENTED_EDGE('',*,*,#1876,.F.);
#2395=ORIENTED_EDGE('',*,*,#1784,.F.);
#2396=ORIENTED_EDGE('',*,*,#1779,.T.);
#2397=ORIENTED_EDGE('',*,*,#1881,.F.);
#2398=ORIENTED_EDGE('',*,*,#1879,.F.);
#2399=ORIENTED_EDGE('',*,*,#1813,.F.);
#2400=ORIENTED_EDGE('',*,*,#1882,.T.);
#2401=ORIENTED_EDGE('',*,*,#1883,.F.);
#2402=ORIENTED_EDGE('',*,*,#1782,.F.);
#2403=ORIENTED_EDGE('',*,*,#1812,.F.);
#2404=ORIENTED_EDGE('',*,*,#1884,.T.);
#2405=ORIENTED_EDGE('',*,*,#1885,.F.);
#2406=ORIENTED_EDGE('',*,*,#1882,.F.);
#2407=ORIENTED_EDGE('',*,*,#1811,.F.);
#2408=ORIENTED_EDGE('',*,*,#1886,.T.);
#2409=ORIENTED_EDGE('',*,*,#1887,.F.);
#2410=ORIENTED_EDGE('',*,*,#1884,.F.);
#2411=ORIENTED_EDGE('',*,*,#1810,.F.);
#2412=ORIENTED_EDGE('',*,*,#1888,.F.);
#2413=ORIENTED_EDGE('',*,*,#1889,.F.);
#2414=ORIENTED_EDGE('',*,*,#1886,.F.);
#2415=ORIENTED_EDGE('',*,*,#1770,.T.);
#2416=ORIENTED_EDGE('',*,*,#1815,.F.);
#2417=ORIENTED_EDGE('',*,*,#1890,.T.);
#2418=ORIENTED_EDGE('',*,*,#1891,.F.);
#2419=ORIENTED_EDGE('',*,*,#1890,.F.);
#2420=ORIENTED_EDGE('',*,*,#1814,.F.);
#2421=ORIENTED_EDGE('',*,*,#1752,.T.);
#2422=ORIENTED_EDGE('',*,*,#1760,.T.);
#2423=ORIENTED_EDGE('',*,*,#1832,.T.);
#2424=ORIENTED_EDGE('',*,*,#1788,.T.);
#2425=ORIENTED_EDGE('',*,*,#1892,.T.);
#2426=ORIENTED_EDGE('',*,*,#1893,.F.);
#2427=ORIENTED_EDGE('',*,*,#1819,.T.);
#2428=ORIENTED_EDGE('',*,*,#1894,.F.);
#2429=ORIENTED_EDGE('',*,*,#1895,.F.);
#2430=ORIENTED_EDGE('',*,*,#1896,.T.);
#2431=ORIENTED_EDGE('',*,*,#1855,.T.);
#2432=ORIENTED_EDGE('',*,*,#1897,.T.);
#2433=ORIENTED_EDGE('',*,*,#1895,.T.);
#2434=ORIENTED_EDGE('',*,*,#1898,.F.);
#2435=ORIENTED_EDGE('',*,*,#1836,.T.);
#2436=ORIENTED_EDGE('',*,*,#1899,.F.);
#2437=ORIENTED_EDGE('',*,*,#1900,.F.);
#2438=ORIENTED_EDGE('',*,*,#1797,.T.);
#2439=ORIENTED_EDGE('',*,*,#1874,.T.);
#2440=ORIENTED_EDGE('',*,*,#1798,.T.);
#2441=ORIENTED_EDGE('',*,*,#1900,.T.);
#2442=ORIENTED_EDGE('',*,*,#1901,.F.);
#2443=ORIENTED_EDGE('',*,*,#1859,.T.);
#2444=ORIENTED_EDGE('',*,*,#1902,.F.);
#2445=ORIENTED_EDGE('',*,*,#1903,.F.);
#2446=ORIENTED_EDGE('',*,*,#1808,.T.);
#2447=ORIENTED_EDGE('',*,*,#1888,.T.);
#2448=ORIENTED_EDGE('',*,*,#1809,.T.);
#2449=ORIENTED_EDGE('',*,*,#1903,.T.);
#2450=ORIENTED_EDGE('',*,*,#1904,.F.);
#2451=ORIENTED_EDGE('',*,*,#1878,.T.);
#2452=ORIENTED_EDGE('',*,*,#1905,.F.);
#2453=ORIENTED_EDGE('',*,*,#1892,.F.);
#2454=ORIENTED_EDGE('',*,*,#1787,.T.);
#2455=ORIENTED_EDGE('',*,*,#1818,.T.);
#2456=ORIENTED_EDGE('',*,*,#1822,.T.);
#2457=ORIENTED_EDGE('',*,*,#1825,.T.);
#2458=ORIENTED_EDGE('',*,*,#1826,.T.);
#2459=ORIENTED_EDGE('',*,*,#1772,.T.);
#2460=ORIENTED_EDGE('',*,*,#1776,.T.);
#2461=ORIENTED_EDGE('',*,*,#1829,.T.);
#2462=ORIENTED_EDGE('',*,*,#1831,.T.);
#2463=ORIENTED_EDGE('',*,*,#1833,.T.);
#2464=ORIENTED_EDGE('',*,*,#1893,.T.);
#2465=ORIENTED_EDGE('',*,*,#1905,.T.);
#2466=ORIENTED_EDGE('',*,*,#1877,.T.);
#2467=ORIENTED_EDGE('',*,*,#1880,.T.);
#2468=ORIENTED_EDGE('',*,*,#1881,.T.);
#2469=ORIENTED_EDGE('',*,*,#1778,.T.);
#2470=ORIENTED_EDGE('',*,*,#1783,.T.);
#2471=ORIENTED_EDGE('',*,*,#1883,.T.);
#2472=ORIENTED_EDGE('',*,*,#1885,.T.);
#2473=ORIENTED_EDGE('',*,*,#1887,.T.);
#2474=ORIENTED_EDGE('',*,*,#1889,.T.);
#2475=ORIENTED_EDGE('',*,*,#1904,.T.);
#2476=ORIENTED_EDGE('',*,*,#1902,.T.);
#2477=ORIENTED_EDGE('',*,*,#1858,.T.);
#2478=ORIENTED_EDGE('',*,*,#1861,.T.);
#2479=ORIENTED_EDGE('',*,*,#1863,.T.);
#2480=ORIENTED_EDGE('',*,*,#1865,.T.);
#2481=ORIENTED_EDGE('',*,*,#1867,.T.);
#2482=ORIENTED_EDGE('',*,*,#1869,.T.);
#2483=ORIENTED_EDGE('',*,*,#1871,.T.);
#2484=ORIENTED_EDGE('',*,*,#1873,.T.);
#2485=ORIENTED_EDGE('',*,*,#1875,.T.);
#2486=ORIENTED_EDGE('',*,*,#1901,.T.);
#2487=ORIENTED_EDGE('',*,*,#1899,.T.);
#2488=ORIENTED_EDGE('',*,*,#1835,.T.);
#2489=ORIENTED_EDGE('',*,*,#1838,.T.);
#2490=ORIENTED_EDGE('',*,*,#1840,.T.);
#2491=ORIENTED_EDGE('',*,*,#1842,.T.);
#2492=ORIENTED_EDGE('',*,*,#1844,.T.);
#2493=ORIENTED_EDGE('',*,*,#1847,.T.);
#2494=ORIENTED_EDGE('',*,*,#1850,.T.);
#2495=ORIENTED_EDGE('',*,*,#1853,.T.);
#2496=ORIENTED_EDGE('',*,*,#1856,.T.);
#2497=ORIENTED_EDGE('',*,*,#1898,.T.);
#2498=ORIENTED_EDGE('',*,*,#1894,.T.);
#2499=ORIENTED_EDGE('',*,*,#1891,.T.);
#2500=ORIENTED_EDGE('',*,*,#1767,.T.);
#2501=ORIENTED_EDGE('',*,*,#1827,.T.);
#2502=ORIENTED_EDGE('',*,*,#1823,.T.);
#2503=ORIENTED_EDGE('',*,*,#1820,.T.);
#2504=ORIENTED_EDGE('',*,*,#1816,.T.);
#2505=ORIENTED_EDGE('',*,*,#1896,.F.);
#2506=ORIENTED_EDGE('',*,*,#1897,.F.);
#2507=ORIENTED_EDGE('',*,*,#1854,.T.);
#2508=ORIENTED_EDGE('',*,*,#1851,.T.);
#2509=ORIENTED_EDGE('',*,*,#1848,.T.);
#2510=ORIENTED_EDGE('',*,*,#1845,.T.);
#2511=ORIENTED_EDGE('',*,*,#1756,.T.);
#3007=CYLINDRICAL_SURFACE('',#3349,0.5);
#3008=CYLINDRICAL_SURFACE('',#3399,0.21);
#3040=ADVANCED_FACE('',(#346),#207,.F.);
#3041=ADVANCED_FACE('',(#347),#208,.T.);
#3042=ADVANCED_FACE('',(#348),#3007,.F.);
#3043=ADVANCED_FACE('',(#349),#209,.F.);
#3044=ADVANCED_FACE('',(#350),#210,.T.);
#3045=ADVANCED_FACE('',(#351),#211,.F.);
#3046=ADVANCED_FACE('',(#352),#212,.F.);
#3047=ADVANCED_FACE('',(#353),#213,.F.);
#3048=ADVANCED_FACE('',(#354),#214,.F.);
#3049=ADVANCED_FACE('',(#355),#215,.F.);
#3050=ADVANCED_FACE('',(#356),#216,.F.);
#3051=ADVANCED_FACE('',(#357),#217,.F.);
#3052=ADVANCED_FACE('',(#358),#218,.F.);
#3053=ADVANCED_FACE('',(#359),#219,.F.);
#3054=ADVANCED_FACE('',(#360),#220,.F.);
#3055=ADVANCED_FACE('',(#361),#221,.F.);
#3056=ADVANCED_FACE('',(#362),#222,.F.);
#3057=ADVANCED_FACE('',(#363),#223,.F.);
#3058=ADVANCED_FACE('',(#364),#224,.F.);
#3059=ADVANCED_FACE('',(#365),#225,.F.);
#3060=ADVANCED_FACE('',(#366),#226,.F.);
#3061=ADVANCED_FACE('',(#367),#227,.F.);
#3062=ADVANCED_FACE('',(#368),#228,.F.);
#3063=ADVANCED_FACE('',(#369),#229,.F.);
#3064=ADVANCED_FACE('',(#370),#230,.F.);
#3065=ADVANCED_FACE('',(#371),#231,.F.);
#3066=ADVANCED_FACE('',(#372),#232,.F.);
#3067=ADVANCED_FACE('',(#373),#233,.F.);
#3068=ADVANCED_FACE('',(#374),#234,.F.);
#3069=ADVANCED_FACE('',(#375),#235,.F.);
#3070=ADVANCED_FACE('',(#376),#236,.F.);
#3071=ADVANCED_FACE('',(#377),#237,.F.);
#3072=ADVANCED_FACE('',(#378),#238,.F.);
#3073=ADVANCED_FACE('',(#379),#239,.F.);
#3074=ADVANCED_FACE('',(#380),#240,.F.);
#3075=ADVANCED_FACE('',(#381),#241,.F.);
#3076=ADVANCED_FACE('',(#382),#242,.F.);
#3077=ADVANCED_FACE('',(#383),#243,.F.);
#3078=ADVANCED_FACE('',(#384),#244,.F.);
#3079=ADVANCED_FACE('',(#385),#245,.F.);
#3080=ADVANCED_FACE('',(#386),#246,.F.);
#3081=ADVANCED_FACE('',(#387),#247,.F.);
#3082=ADVANCED_FACE('',(#388),#248,.F.);
#3083=ADVANCED_FACE('',(#389),#3008,.F.);
#3084=ADVANCED_FACE('',(#390),#249,.T.);
#3085=ADVANCED_FACE('',(#391),#250,.T.);
#3086=ADVANCED_FACE('',(#392),#251,.T.);
#3087=ADVANCED_FACE('',(#393),#252,.T.);
#3088=ADVANCED_FACE('',(#394),#253,.T.);
#3089=ADVANCED_FACE('',(#395),#254,.T.);
#3090=ADVANCED_FACE('',(#396),#255,.T.);
#3091=ADVANCED_FACE('',(#397),#256,.T.);
#3092=ADVANCED_FACE('',(#398,#183),#257,.T.);
#3093=ADVANCED_FACE('',(#399),#258,.F.);
#3206=CLOSED_SHELL('',(#3040,#3041,#3042,#3043,#3044,#3045,#3046,#3047,
#3048,#3049,#3050,#3051,#3052,#3053,#3054,#3055,#3056,#3057,#3058,#3059,
#3060,#3061,#3062,#3063,#3064,#3065,#3066,#3067,#3068,#3069,#3070,#3071,
#3072,#3073,#3074,#3075,#3076,#3077,#3078,#3079,#3080,#3081,#3082,#3083,
#3084,#3085,#3086,#3087,#3088,#3089,#3090,#3091,#3092,#3093));
#3344=AXIS2_PLACEMENT_3D('',#4577,#3667,#3668);
#3345=AXIS2_PLACEMENT_3D('',#4578,#3669,#3670);
#3346=AXIS2_PLACEMENT_3D('',#4583,#3672,#3673);
#3347=AXIS2_PLACEMENT_3D('',#4585,#3675,#3676);
#3348=AXIS2_PLACEMENT_3D('',#4590,#3678,#3679);
#3349=AXIS2_PLACEMENT_3D('',#4594,#3682,#3683);
#3350=AXIS2_PLACEMENT_3D('',#4597,#3684,#3685);
#3351=AXIS2_PLACEMENT_3D('',#4599,#3686,#3687);
#3352=AXIS2_PLACEMENT_3D('',#4603,#3689,#3690);
#3353=AXIS2_PLACEMENT_3D('',#4607,#3692,#3693);
#3354=AXIS2_PLACEMENT_3D('',#4617,#3695,#3696);
#3355=AXIS2_PLACEMENT_3D('',#4620,#3698,#3699);
#3356=AXIS2_PLACEMENT_3D('',#4621,#3700,#3701);
#3357=AXIS2_PLACEMENT_3D('',#4622,#3702,#3703);
#3358=AXIS2_PLACEMENT_3D('',#4626,#3706,#3707);
#3359=AXIS2_PLACEMENT_3D('',#4632,#3711,#3712);
#3360=AXIS2_PLACEMENT_3D('',#4638,#3716,#3717);
#3361=AXIS2_PLACEMENT_3D('',#4644,#3721,#3722);
#3362=AXIS2_PLACEMENT_3D('',#4652,#3727,#3728);
#3363=AXIS2_PLACEMENT_3D('',#4658,#3732,#3733);
#3364=AXIS2_PLACEMENT_3D('',#4674,#3742,#3743);
#3365=AXIS2_PLACEMENT_3D('',#4719,#3766,#3767);
#3366=AXIS2_PLACEMENT_3D('',#4720,#3768,#3769);
#3367=AXIS2_PLACEMENT_3D('',#4721,#3770,#3771);
#3368=AXIS2_PLACEMENT_3D('',#4730,#3776,#3777);
#3369=AXIS2_PLACEMENT_3D('',#4736,#3781,#3782);
#3370=AXIS2_PLACEMENT_3D('',#4742,#3786,#3787);
#3371=AXIS2_PLACEMENT_3D('',#4745,#3790,#3791);
#3372=AXIS2_PLACEMENT_3D('',#4749,#3794,#3795);
#3373=AXIS2_PLACEMENT_3D('',#4753,#3798,#3799);
#3374=AXIS2_PLACEMENT_3D('',#4757,#3802,#3803);
#3375=AXIS2_PLACEMENT_3D('',#4763,#3807,#3808);
#3376=AXIS2_PLACEMENT_3D('',#4767,#3811,#3812);
#3377=AXIS2_PLACEMENT_3D('',#4771,#3815,#3816);
#3378=AXIS2_PLACEMENT_3D('',#4775,#3819,#3820);
#3379=AXIS2_PLACEMENT_3D('',#4779,#3823,#3824);
#3380=AXIS2_PLACEMENT_3D('',#4785,#3828,#3829);
#3381=AXIS2_PLACEMENT_3D('',#4791,#3833,#3834);
#3382=AXIS2_PLACEMENT_3D('',#4797,#3838,#3839);
#3383=AXIS2_PLACEMENT_3D('',#4803,#3843,#3844);
#3384=AXIS2_PLACEMENT_3D('',#4809,#3848,#3849);
#3385=AXIS2_PLACEMENT_3D('',#4813,#3852,#3853);
#3386=AXIS2_PLACEMENT_3D('',#4817,#3856,#3857);
#3387=AXIS2_PLACEMENT_3D('',#4821,#3860,#3861);
#3388=AXIS2_PLACEMENT_3D('',#4825,#3864,#3865);
#3389=AXIS2_PLACEMENT_3D('',#4829,#3868,#3869);
#3390=AXIS2_PLACEMENT_3D('',#4833,#3872,#3873);
#3391=AXIS2_PLACEMENT_3D('',#4837,#3876,#3877);
#3392=AXIS2_PLACEMENT_3D('',#4841,#3880,#3881);
#3393=AXIS2_PLACEMENT_3D('',#4847,#3885,#3886);
#3394=AXIS2_PLACEMENT_3D('',#4851,#3889,#3890);
#3395=AXIS2_PLACEMENT_3D('',#4853,#3892,#3893);
#3396=AXIS2_PLACEMENT_3D('',#4857,#3896,#3897);
#3397=AXIS2_PLACEMENT_3D('',#4861,#3900,#3901);
#3398=AXIS2_PLACEMENT_3D('',#4865,#3904,#3905);
#3399=AXIS2_PLACEMENT_3D('',#4869,#3908,#3909);
#3400=AXIS2_PLACEMENT_3D('',#4872,#3911,#3912);
#3401=AXIS2_PLACEMENT_3D('',#4873,#3913,#3914);
#3402=AXIS2_PLACEMENT_3D('',#4877,#3917,#3918);
#3403=AXIS2_PLACEMENT_3D('',#4883,#3922,#3923);
#3404=AXIS2_PLACEMENT_3D('',#4886,#3926,#3927);
#3405=AXIS2_PLACEMENT_3D('',#4890,#3930,#3931);
#3406=AXIS2_PLACEMENT_3D('',#4892,#3933,#3934);
#3407=AXIS2_PLACEMENT_3D('',#4896,#3937,#3938);
#3408=AXIS2_PLACEMENT_3D('',#4898,#3940,#3941);
#3409=AXIS2_PLACEMENT_3D('',#4900,#3943,#3944);
#3410=AXIS2_PLACEMENT_3D('',#4901,#3945,#3946);
#3667=DIRECTION('axis',(0.,0.,1.));
#3668=DIRECTION('refdir',(1.,0.,0.));
#3669=DIRECTION('center_axis',(0.,1.,0.));
#3670=DIRECTION('ref_axis',(1.,0.,0.));
#3671=DIRECTION('',(-1.,0.,0.));
#3672=DIRECTION('center_axis',(0.,1.,0.));
#3673=DIRECTION('ref_axis',(1.,0.,0.));
#3674=DIRECTION('',(0.,0.,1.));
#3675=DIRECTION('center_axis',(0.,1.,0.));
#3676=DIRECTION('ref_axis',(1.,0.,0.));
#3677=DIRECTION('',(-1.,0.,0.));
#3678=DIRECTION('center_axis',(0.,1.,0.));
#3679=DIRECTION('ref_axis',(1.,0.,0.));
#3680=DIRECTION('',(1.,0.,0.));
#3681=DIRECTION('',(0.,0.,-1.));
#3682=DIRECTION('center_axis',(0.,1.,0.));
#3683=DIRECTION('ref_axis',(1.,0.,0.));
#3684=DIRECTION('center_axis',(0.,-0.707106781186547,-0.707106781186548));
#3685=DIRECTION('ref_axis',(0.,0.707106781186548,-0.707106781186547));
#3686=DIRECTION('center_axis',(0.,1.,0.));
#3687=DIRECTION('ref_axis',(1.,0.,0.));
#3688=DIRECTION('',(0.,1.,0.));
#3689=DIRECTION('center_axis',(0.,0.707106781186548,0.707106781186547));
#3690=DIRECTION('ref_axis',(0.,0.707106781186547,-0.707106781186548));
#3691=DIRECTION('',(0.,1.,0.));
#3692=DIRECTION('center_axis',(0.,1.,0.));
#3693=DIRECTION('ref_axis',(1.,0.,0.));
#3694=DIRECTION('',(0.,-1.,0.));
#3695=DIRECTION('center_axis',(0.,0.707106781186547,-0.707106781186548));
#3696=DIRECTION('ref_axis',(0.,-0.707106781186548,-0.707106781186547));
#3697=DIRECTION('',(0.,-1.,0.));
#3698=DIRECTION('center_axis',(0.,-0.707106781186547,0.707106781186548));
#3699=DIRECTION('ref_axis',(0.,-0.707106781186548,-0.707106781186547));
#3700=DIRECTION('center_axis',(0.,-1.,2.77555756156289E-16));
#3701=DIRECTION('ref_axis',(1.,0.,0.));
#3702=DIRECTION('center_axis',(0.,1.,0.));
#3703=DIRECTION('ref_axis',(1.,0.,0.));
#3704=DIRECTION('',(1.,0.,0.));
#3705=DIRECTION('',(0.,0.,1.));
#3706=DIRECTION('center_axis',(0.,1.,0.));
#3707=DIRECTION('ref_axis',(1.,0.,0.));
#3708=DIRECTION('',(1.,0.,0.));
#3709=DIRECTION('',(0.,0.,-1.));
#3710=DIRECTION('',(-1.,0.,0.));
#3711=DIRECTION('center_axis',(0.,-1.,2.77555756156289E-16));
#3712=DIRECTION('ref_axis',(0.,-2.77555756156289E-16,-1.));
#3713=DIRECTION('',(1.,0.,0.));
#3714=DIRECTION('',(0.,2.77555756156289E-16,1.));
#3715=DIRECTION('',(1.,0.,0.));
#3716=DIRECTION('center_axis',(0.,-0.707106781186547,0.707106781186548));
#3717=DIRECTION('ref_axis',(0.,-0.707106781186548,-0.707106781186547));
#3718=DIRECTION('',(0.,-0.707106781186548,-0.707106781186547));
#3719=DIRECTION('',(1.,0.,0.));
#3720=DIRECTION('',(0.,0.707106781186548,0.707106781186547));
#3721=DIRECTION('center_axis',(0.,0.707106781186547,-0.707106781186548));
#3722=DIRECTION('ref_axis',(0.,0.707106781186548,0.707106781186547));
#3723=DIRECTION('',(1.,0.,0.));
#3724=DIRECTION('',(0.,-0.707106781186548,-0.707106781186547));
#3725=DIRECTION('',(1.,0.,0.));
#3726=DIRECTION('',(0.,0.707106781186548,0.707106781186547));
#3727=DIRECTION('center_axis',(0.,0.,-1.));
#3728=DIRECTION('ref_axis',(0.,1.,0.));
#3729=DIRECTION('',(0.,1.,0.));
#3730=DIRECTION('',(1.,0.,0.));
#3731=DIRECTION('',(0.,-1.,0.));
#3732=DIRECTION('center_axis',(1.,0.,0.));
#3733=DIRECTION('ref_axis',(0.,0.,-1.));
#3734=DIRECTION('',(0.,0.,1.));
#3735=DIRECTION('',(0.,-1.,0.));
#3736=DIRECTION('',(0.,0.,1.));
#3737=DIRECTION('',(0.,-1.,0.));
#3738=DIRECTION('',(0.,0.,1.));
#3739=DIRECTION('',(0.,-1.,2.41352831440251E-16));
#3740=DIRECTION('',(0.,4.44089209850063E-16,1.));
#3741=DIRECTION('',(0.,-1.,7.40148683083438E-16));
#3742=DIRECTION('center_axis',(1.,0.,0.));
#3743=DIRECTION('ref_axis',(0.,0.,-1.));
#3744=DIRECTION('',(0.,-1.,0.));
#3745=DIRECTION('',(0.,-0.707106781186548,-0.707106781186547));
#3746=DIRECTION('',(0.,0.,-1.));
#3747=DIRECTION('',(0.,1.,0.));
#3748=DIRECTION('',(0.,-2.41352831440251E-16,-1.));
#3749=DIRECTION('',(0.,1.,0.));
#3750=DIRECTION('',(0.,0.,-1.));
#3751=DIRECTION('',(0.,1.,0.));
#3752=DIRECTION('',(0.,0.,-1.));
#3753=DIRECTION('',(0.,1.,-7.40148683083438E-16));
#3754=DIRECTION('',(0.,0.707106781186547,0.707106781186548));
#3755=DIRECTION('',(0.,0.,1.));
#3756=DIRECTION('',(0.,-0.707106781186548,0.707106781186548));
#3757=DIRECTION('',(0.,-1.,0.));
#3758=DIRECTION('',(0.,0.,-1.));
#3759=DIRECTION('',(0.,-1.,0.));
#3760=DIRECTION('',(0.,0.,-1.));
#3761=DIRECTION('',(0.,-1.,0.));
#3762=DIRECTION('',(0.,0.,-1.));
#3763=DIRECTION('',(0.,-1.,0.));
#3764=DIRECTION('',(0.,0.,-1.));
#3765=DIRECTION('',(0.,0.707106781186548,-0.707106781186547));
#3766=DIRECTION('center_axis',(1.,0.,0.));
#3767=DIRECTION('ref_axis',(0.,0.,-1.));
#3768=DIRECTION('center_axis',(1.,0.,0.));
#3769=DIRECTION('ref_axis',(0.,0.,-1.));
#3770=DIRECTION('center_axis',(0.,0.,-1.));
#3771=DIRECTION('ref_axis',(0.,1.,0.));
#3772=DIRECTION('',(0.,1.,0.));
#3773=DIRECTION('',(1.,0.,0.));
#3774=DIRECTION('',(0.,-1.,0.));
#3775=DIRECTION('',(1.,0.,0.));
#3776=DIRECTION('center_axis',(0.,1.,-8.88178419700125E-16));
#3777=DIRECTION('ref_axis',(0.,8.88178419700125E-16,1.));
#3778=DIRECTION('',(0.,8.88178419700125E-16,1.));
#3779=DIRECTION('',(1.,0.,0.));
#3780=DIRECTION('',(0.,-8.88178419700125E-16,-1.));
#3781=DIRECTION('center_axis',(0.,-7.40148683083439E-16,-1.));
#3782=DIRECTION('ref_axis',(0.,1.,-7.40148683083439E-16));
#3783=DIRECTION('',(0.,1.,-7.40148683083439E-16));
#3784=DIRECTION('',(1.,0.,0.));
#3785=DIRECTION('',(0.,-1.,7.40148683083439E-16));
#3786=DIRECTION('center_axis',(0.,-0.707106781186547,-0.707106781186548));
#3787=DIRECTION('ref_axis',(0.,0.707106781186548,-0.707106781186547));
#3788=DIRECTION('',(0.,-0.707106781186548,0.707106781186547));
#3789=DIRECTION('',(0.,0.707106781186548,-0.707106781186547));
#3790=DIRECTION('center_axis',(0.,7.40148683083438E-16,1.));
#3791=DIRECTION('ref_axis',(0.,-1.,7.40148683083438E-16));
#3792=DIRECTION('',(1.,0.,0.));
#3793=DIRECTION('',(0.,1.,-7.40148683083438E-16));
#3794=DIRECTION('center_axis',(0.,1.,-4.44089209850063E-16));
#3795=DIRECTION('ref_axis',(0.,4.44089209850063E-16,1.));
#3796=DIRECTION('',(1.,0.,0.));
#3797=DIRECTION('',(0.,-4.44089209850063E-16,-1.));
#3798=DIRECTION('center_axis',(0.,2.41352831440251E-16,1.));
#3799=DIRECTION('ref_axis',(0.,-1.,2.41352831440251E-16));
#3800=DIRECTION('',(-1.,0.,0.));
#3801=DIRECTION('',(0.,1.,-2.41352831440251E-16));
#3802=DIRECTION('center_axis',(0.,-1.,2.41352831440251E-16));
#3803=DIRECTION('ref_axis',(0.,-2.41352831440251E-16,-1.));
#3804=DIRECTION('',(1.,0.,0.));
#3805=DIRECTION('',(0.,2.41352831440251E-16,1.));
#3806=DIRECTION('',(1.,0.,0.));
#3807=DIRECTION('center_axis',(0.,0.,-1.));
#3808=DIRECTION('ref_axis',(0.,1.,0.));
#3809=DIRECTION('',(1.,0.,0.));
#3810=DIRECTION('',(0.,-1.,0.));
#3811=DIRECTION('center_axis',(0.,-1.,0.));
#3812=DIRECTION('ref_axis',(0.,0.,-1.));
#3813=DIRECTION('',(1.,0.,0.));
#3814=DIRECTION('',(0.,0.,1.));
#3815=DIRECTION('center_axis',(0.,-0.707106781186547,0.707106781186548));
#3816=DIRECTION('ref_axis',(0.,-0.707106781186548,-0.707106781186547));
#3817=DIRECTION('',(1.,0.,0.));
#3818=DIRECTION('',(0.,0.707106781186548,0.707106781186547));
#3819=DIRECTION('center_axis',(0.,0.,1.));
#3820=DIRECTION('ref_axis',(0.,-1.,0.));
#3821=DIRECTION('',(1.,0.,0.));
#3822=DIRECTION('',(0.,1.,0.));
#3823=DIRECTION('center_axis',(0.,0.707106781186548,0.707106781186547));
#3824=DIRECTION('ref_axis',(0.,-0.707106781186547,0.707106781186548));
#3825=DIRECTION('',(0.,-0.707106781186547,0.707106781186548));
#3826=DIRECTION('',(1.,0.,0.));
#3827=DIRECTION('',(0.,0.707106781186547,-0.707106781186548));
#3828=DIRECTION('center_axis',(0.,1.,0.));
#3829=DIRECTION('ref_axis',(0.,0.,1.));
#3830=DIRECTION('',(0.,0.,1.));
#3831=DIRECTION('',(1.,0.,0.));
#3832=DIRECTION('',(0.,0.,-1.));
#3833=DIRECTION('center_axis',(0.,0.,-1.));
#3834=DIRECTION('ref_axis',(0.,1.,0.));
#3835=DIRECTION('',(0.,1.,0.));
#3836=DIRECTION('',(1.,0.,0.));
#3837=DIRECTION('',(0.,-1.,0.));
#3838=DIRECTION('center_axis',(0.,1.,-2.41352831440251E-16));
#3839=DIRECTION('ref_axis',(0.,2.41352831440251E-16,1.));
#3840=DIRECTION('',(0.,2.41352831440251E-16,1.));
#3841=DIRECTION('',(-1.,0.,0.));
#3842=DIRECTION('',(0.,-2.41352831440251E-16,-1.));
#3843=DIRECTION('center_axis',(0.,0.,1.));
#3844=DIRECTION('ref_axis',(0.,-1.,0.));
#3845=DIRECTION('',(1.,0.,0.));
#3846=DIRECTION('',(0.,1.,0.));
#3847=DIRECTION('',(1.,0.,0.));
#3848=DIRECTION('center_axis',(0.,-1.,0.));
#3849=DIRECTION('ref_axis',(0.,0.,-1.));
#3850=DIRECTION('',(1.,0.,0.));
#3851=DIRECTION('',(0.,0.,1.));
#3852=DIRECTION('center_axis',(0.,0.,1.));
#3853=DIRECTION('ref_axis',(0.,-1.,0.));
#3854=DIRECTION('',(1.,0.,0.));
#3855=DIRECTION('',(0.,1.,0.));
#3856=DIRECTION('center_axis',(0.,0.707106781186548,0.707106781186548));
#3857=DIRECTION('ref_axis',(0.,-0.707106781186548,0.707106781186548));
#3858=DIRECTION('',(1.,0.,0.));
#3859=DIRECTION('',(0.,0.707106781186548,-0.707106781186548));
#3860=DIRECTION('center_axis',(0.,1.,0.));
#3861=DIRECTION('ref_axis',(0.,0.,1.));
#3862=DIRECTION('',(1.,0.,0.));
#3863=DIRECTION('',(0.,0.,-1.));
#3864=DIRECTION('center_axis',(0.,0.707106781186548,-0.707106781186547));
#3865=DIRECTION('ref_axis',(0.,0.707106781186547,0.707106781186548));
#3866=DIRECTION('',(1.,0.,0.));
#3867=DIRECTION('',(0.,-0.707106781186547,-0.707106781186548));
#3868=DIRECTION('center_axis',(0.,-7.40148683083438E-16,-1.));
#3869=DIRECTION('ref_axis',(0.,1.,-7.40148683083438E-16));
#3870=DIRECTION('',(1.,0.,0.));
#3871=DIRECTION('',(0.,-1.,7.40148683083438E-16));
#3872=DIRECTION('center_axis',(0.,-1.,0.));
#3873=DIRECTION('ref_axis',(0.,0.,-1.));
#3874=DIRECTION('',(1.,0.,0.));
#3875=DIRECTION('',(0.,0.,1.));
#3876=DIRECTION('center_axis',(0.,0.,-1.));
#3877=DIRECTION('ref_axis',(0.,1.,0.));
#3878=DIRECTION('',(-1.,0.,0.));
#3879=DIRECTION('',(0.,-1.,0.));
#3880=DIRECTION('center_axis',(0.,1.,0.));
#3881=DIRECTION('ref_axis',(0.,0.,1.));
#3882=DIRECTION('',(1.,0.,0.));
#3883=DIRECTION('',(0.,0.,-1.));
#3884=DIRECTION('',(1.,0.,0.));
#3885=DIRECTION('center_axis',(0.,0.,1.));
#3886=DIRECTION('ref_axis',(0.,-1.,0.));
#3887=DIRECTION('',(1.,0.,0.));
#3888=DIRECTION('',(0.,1.,0.));
#3889=DIRECTION('center_axis',(0.,1.,0.));
#3890=DIRECTION('ref_axis',(0.,0.,1.));
#3891=DIRECTION('',(0.,0.,-1.));
#3892=DIRECTION('center_axis',(0.,-0.707106781186547,-0.707106781186548));
#3893=DIRECTION('ref_axis',(0.,0.707106781186548,-0.707106781186547));
#3894=DIRECTION('',(1.,0.,0.));
#3895=DIRECTION('',(0.,-0.707106781186548,0.707106781186547));
#3896=DIRECTION('center_axis',(0.,-1.,0.));
#3897=DIRECTION('ref_axis',(0.,0.,-1.));
#3898=DIRECTION('',(1.,0.,0.));
#3899=DIRECTION('',(0.,0.,1.));
#3900=DIRECTION('center_axis',(0.,0.,1.));
#3901=DIRECTION('ref_axis',(0.,-1.,0.));
#3902=DIRECTION('',(1.,0.,0.));
#3903=DIRECTION('',(0.,1.,0.));
#3904=DIRECTION('center_axis',(0.,-1.,0.));
#3905=DIRECTION('ref_axis',(0.,0.,-1.));
#3906=DIRECTION('',(-1.,0.,0.));
#3907=DIRECTION('',(0.,0.,1.));
#3908=DIRECTION('center_axis',(1.,0.,0.));
#3909=DIRECTION('ref_axis',(0.,0.,-1.));
#3910=DIRECTION('',(1.,0.,0.));
#3911=DIRECTION('center_axis',(-1.,0.,0.));
#3912=DIRECTION('ref_axis',(0.,0.,-1.));
#3913=DIRECTION('center_axis',(0.,1.,0.));
#3914=DIRECTION('ref_axis',(0.,0.,1.));
#3915=DIRECTION('',(1.,0.,0.));
#3916=DIRECTION('',(0.,0.,1.));
#3917=DIRECTION('center_axis',(0.,1.,0.));
#3918=DIRECTION('ref_axis',(0.,0.,1.));
#3919=DIRECTION('',(0.,0.,1.));
#3920=DIRECTION('',(1.,0.,0.));
#3921=DIRECTION('',(0.,0.,1.));
#3922=DIRECTION('center_axis',(0.,0.,-1.));
#3923=DIRECTION('ref_axis',(0.,1.,0.));
#3924=DIRECTION('',(0.,1.,0.));
#3925=DIRECTION('',(0.,1.,0.));
#3926=DIRECTION('center_axis',(0.,0.,-1.));
#3927=DIRECTION('ref_axis',(0.,1.,0.));
#3928=DIRECTION('',(0.,1.,0.));
#3929=DIRECTION('',(1.,0.,0.));
#3930=DIRECTION('center_axis',(0.,-1.,0.));
#3931=DIRECTION('ref_axis',(0.,0.,-1.));
#3932=DIRECTION('',(0.,0.,-1.));
#3933=DIRECTION('center_axis',(0.,-1.,0.));
#3934=DIRECTION('ref_axis',(0.,0.,-1.));
#3935=DIRECTION('',(0.,0.,-1.));
#3936=DIRECTION('',(1.,0.,0.));
#3937=DIRECTION('center_axis',(0.,0.,1.));
#3938=DIRECTION('ref_axis',(0.,-1.,0.));
#3939=DIRECTION('',(0.,-1.,0.));
#3940=DIRECTION('center_axis',(0.,0.,1.));
#3941=DIRECTION('ref_axis',(0.,-1.,0.));
#3942=DIRECTION('',(0.,-1.,0.));
#3943=DIRECTION('center_axis',(1.,0.,0.));
#3944=DIRECTION('ref_axis',(0.,0.,-1.));
#3945=DIRECTION('center_axis',(1.,0.,0.));
#3946=DIRECTION('ref_axis',(0.,0.,-1.));
#4577=CARTESIAN_POINT('',(0.,0.,0.));
#4578=CARTESIAN_POINT('Origin',(0.,0.6,0.));
#4579=CARTESIAN_POINT('',(0.14,0.6,0.48));
#4580=CARTESIAN_POINT('',(6.93889390390723E-18,0.6,0.48));
#4581=CARTESIAN_POINT('',(-0.05,0.6,0.48));
#4582=CARTESIAN_POINT('',(0.,0.6,0.5));
#4583=CARTESIAN_POINT('Origin',(0.,0.6,0.));
#4584=CARTESIAN_POINT('',(0.,0.6,0.));
#4585=CARTESIAN_POINT('Origin',(0.,0.2,0.));
#4586=CARTESIAN_POINT('',(0.271293199325011,0.2,0.42));
#4587=CARTESIAN_POINT('',(0.,0.2,0.42));
#4588=CARTESIAN_POINT('',(-0.05,0.2,0.42));
#4589=CARTESIAN_POINT('',(0.495883050728698,0.2,0.0640312423743282));
#4590=CARTESIAN_POINT('Origin',(0.,0.2,0.));
#4591=CARTESIAN_POINT('',(0.,0.2,0.0640312423743285));
#4592=CARTESIAN_POINT('',(-0.1,0.2,0.0640312423743285));
#4593=CARTESIAN_POINT('',(0.,0.2,0.));
#4594=CARTESIAN_POINT('Origin',(0.,0.2,0.));
#4595=CARTESIAN_POINT('',(0.139999999999999,0.6,-0.48));
#4596=CARTESIAN_POINT('',(0.4,0.42,-0.3));
#4597=CARTESIAN_POINT('Origin',(0.,0.12,0.));
#4598=CARTESIAN_POINT('',(0.,0.6,-0.5));
#4599=CARTESIAN_POINT('Origin',(0.,0.6,0.));
#4600=CARTESIAN_POINT('',(0.,0.38,-0.5));
#4601=CARTESIAN_POINT('',(0.,0.2,-0.5));
#4602=CARTESIAN_POINT('',(0.271293199325011,0.3,-0.42));
#4603=CARTESIAN_POINT('Origin',(0.,-0.12,0.));
#4604=CARTESIAN_POINT('',(0.271293199325011,0.2,-0.42));
#4605=CARTESIAN_POINT('',(0.271293199325011,0.2,-0.42));
#4606=CARTESIAN_POINT('',(0.495883050728698,0.2,-0.0640312423743282));
#4607=CARTESIAN_POINT('Origin',(0.,0.2,0.));
#4608=CARTESIAN_POINT('Ctrl Pts',(0.495883050728698,0.2,0.0640312423743283));
#4609=CARTESIAN_POINT('Ctrl Pts',(0.498592889791231,0.206718816306565,0.0430451860136323));
#4610=CARTESIAN_POINT('Ctrl Pts',(0.5,0.21,0.0210250906311155));
#4611=CARTESIAN_POINT('Ctrl Pts',(0.5,0.21,-0.0210250906311155));
#4612=CARTESIAN_POINT('Ctrl Pts',(0.498592889791231,0.206718816306565,-0.0430451860136323));
#4613=CARTESIAN_POINT('Ctrl Pts',(0.495883050728698,0.2,-0.0640312423743282));
#4614=CARTESIAN_POINT('',(0.271293199325011,0.3,0.42));
#4615=CARTESIAN_POINT('',(0.271293199325011,0.2,0.42));
#4616=CARTESIAN_POINT('',(6.93889390390723E-18,0.38,0.5));
#4617=CARTESIAN_POINT('Origin',(0.,-0.12,0.));
#4618=CARTESIAN_POINT('',(0.,0.2,0.5));
#4619=CARTESIAN_POINT('',(0.4,0.42,0.3));
#4620=CARTESIAN_POINT('Origin',(0.,0.12,0.));
#4621=CARTESIAN_POINT('Origin',(0.,0.42,0.));
#4622=CARTESIAN_POINT('Origin',(0.,0.6,0.));
#4623=CARTESIAN_POINT('',(0.,0.6,-0.48));
#4624=CARTESIAN_POINT('',(-0.05,0.6,-0.48));
#4625=CARTESIAN_POINT('',(0.,0.6,0.));
#4626=CARTESIAN_POINT('Origin',(0.,0.2,0.));
#4627=CARTESIAN_POINT('',(0.,0.2,-0.42));
#4628=CARTESIAN_POINT('',(-0.05,0.2,-0.42));
#4629=CARTESIAN_POINT('',(0.,0.2,-0.0640312423743285));
#4630=CARTESIAN_POINT('',(0.,0.2,0.));
#4631=CARTESIAN_POINT('',(-0.1,0.2,-0.0640312423743285));
#4632=CARTESIAN_POINT('Origin',(-0.1,0.42,0.3));
#4633=CARTESIAN_POINT('',(10.,0.42,0.3));
#4634=CARTESIAN_POINT('',(-0.1,0.42,0.3));
#4635=CARTESIAN_POINT('',(10.,0.42,-0.3));
#4636=CARTESIAN_POINT('',(10.,0.42,0.15));
#4637=CARTESIAN_POINT('',(-0.1,0.42,-0.3));
#4638=CARTESIAN_POINT('Origin',(-0.1,0.67,0.55));
#4639=CARTESIAN_POINT('',(0.,0.67,0.55));
#4640=CARTESIAN_POINT('',(6.93889390390723E-18,0.365,0.245));
#4641=CARTESIAN_POINT('',(10.,0.67,0.55));
#4642=CARTESIAN_POINT('',(-0.1,0.67,0.55));
#4643=CARTESIAN_POINT('',(10.,0.365,0.245));
#4644=CARTESIAN_POINT('Origin',(-0.1,0.3,0.42));
#4645=CARTESIAN_POINT('',(10.,0.3,0.42));
#4646=CARTESIAN_POINT('',(-0.1,0.3,0.42));
#4647=CARTESIAN_POINT('',(10.,0.55,0.67));
#4648=CARTESIAN_POINT('',(10.,0.12,0.24));
#4649=CARTESIAN_POINT('',(0.,0.55,0.67));
#4650=CARTESIAN_POINT('',(-0.1,0.55,0.67));
#4651=CARTESIAN_POINT('',(6.93889390390723E-18,0.12,0.24));
#4652=CARTESIAN_POINT('Origin',(-0.1,-0.3,0.42));
#4653=CARTESIAN_POINT('',(0.,-0.3,0.42));
#4654=CARTESIAN_POINT('',(0.,-0.15,0.42));
#4655=CARTESIAN_POINT('',(10.,-0.3,0.42));
#4656=CARTESIAN_POINT('',(-0.1,-0.3,0.42));
#4657=CARTESIAN_POINT('',(10.,-0.15,0.42));
#4658=CARTESIAN_POINT('Origin',(0.,0.,0.));
#4659=CARTESIAN_POINT('',(0.,0.55,0.82));
#4660=CARTESIAN_POINT('',(0.,0.55,0.335));
#4661=CARTESIAN_POINT('',(0.,0.3,0.82));
#4662=CARTESIAN_POINT('',(0.,0.275,0.82));
#4663=CARTESIAN_POINT('',(0.,0.3,1.));
#4664=CARTESIAN_POINT('',(0.,0.3,0.41));
#4665=CARTESIAN_POINT('',(0.,1.,1.));
#4666=CARTESIAN_POINT('',(0.,1.,1.));
#4667=CARTESIAN_POINT('',(0.,1.,0.3));
#4668=CARTESIAN_POINT('',(0.,1.,-1.));
#4669=CARTESIAN_POINT('',(0.,0.82,0.3));
#4670=CARTESIAN_POINT('',(0.,0.525,0.3));
#4671=CARTESIAN_POINT('',(0.,0.82,0.55));
#4672=CARTESIAN_POINT('',(0.,0.82,0.15));
#4673=CARTESIAN_POINT('',(0.,0.41,0.55));
#4674=CARTESIAN_POINT('Origin',(0.,0.,0.));
#4675=CARTESIAN_POINT('',(0.,-0.3,-0.42));
#4676=CARTESIAN_POINT('',(0.,0.15,-0.42));
#4677=CARTESIAN_POINT('',(0.,-0.55,-0.67));
#4678=CARTESIAN_POINT('',(0.,-0.12,-0.24));
#4679=CARTESIAN_POINT('',(0.,-0.55,-0.82));
#4680=CARTESIAN_POINT('',(0.,-0.55,-0.335));
#4681=CARTESIAN_POINT('',(0.,-0.3,-0.82));
#4682=CARTESIAN_POINT('',(0.,-0.275,-0.82));
#4683=CARTESIAN_POINT('',(0.,-0.3,-1.));
#4684=CARTESIAN_POINT('',(0.,-0.3,-0.41));
#4685=CARTESIAN_POINT('',(0.,-1.,-1.));
#4686=CARTESIAN_POINT('',(0.,-1.,-1.));
#4687=CARTESIAN_POINT('',(0.,-1.,-0.3));
#4688=CARTESIAN_POINT('',(0.,-1.,1.));
#4689=CARTESIAN_POINT('',(0.,-0.82,-0.3));
#4690=CARTESIAN_POINT('',(0.,-0.525,-0.3));
#4691=CARTESIAN_POINT('',(0.,-0.82,-0.55));
#4692=CARTESIAN_POINT('',(0.,-0.82,-0.15));
#4693=CARTESIAN_POINT('',(0.,-0.67,-0.55));
#4694=CARTESIAN_POINT('',(0.,-0.41,-0.55));
#4695=CARTESIAN_POINT('',(0.,-0.42,-0.3));
#4696=CARTESIAN_POINT('',(0.,-0.365,-0.245));
#4697=CARTESIAN_POINT('',(0.,-0.42,0.3));
#4698=CARTESIAN_POINT('',(0.,-0.42,-0.15));
#4699=CARTESIAN_POINT('',(0.,-0.67,0.55));
#4700=CARTESIAN_POINT('',(-6.93889390390723E-18,-0.24,0.12));
#4701=CARTESIAN_POINT('',(0.,-0.82,0.55));
#4702=CARTESIAN_POINT('',(0.,-0.335,0.55));
#4703=CARTESIAN_POINT('',(0.,-0.82,0.3));
#4704=CARTESIAN_POINT('',(0.,-0.82,0.275));
#4705=CARTESIAN_POINT('',(0.,-1.,0.3));
#4706=CARTESIAN_POINT('',(0.,-0.41,0.3));
#4707=CARTESIAN_POINT('',(0.,-1.,1.));
#4708=CARTESIAN_POINT('',(0.,-1.,1.));
#4709=CARTESIAN_POINT('',(0.,-0.3,1.));
#4710=CARTESIAN_POINT('',(0.,1.,1.));
#4711=CARTESIAN_POINT('',(0.,-0.3,0.82));
#4712=CARTESIAN_POINT('',(0.,-0.3,0.525));
#4713=CARTESIAN_POINT('',(0.,-0.55,0.82));
#4714=CARTESIAN_POINT('',(0.,-0.15,0.82));
#4715=CARTESIAN_POINT('',(0.,-0.55,0.67));
#4716=CARTESIAN_POINT('',(0.,-0.55,0.41));
#4717=CARTESIAN_POINT('',(6.93889390390723E-18,-0.245,0.365));
#4718=CARTESIAN_POINT('',(0.,-2.57175827820944E-17,0.21));
#4719=CARTESIAN_POINT('Origin',(0.,0.,0.));
#4720=CARTESIAN_POINT('Origin',(0.,0.,0.));
#4721=CARTESIAN_POINT('Origin',(-0.1,0.82,-0.3));
#4722=CARTESIAN_POINT('',(0.,0.82,-0.3));
#4723=CARTESIAN_POINT('',(0.,1.,-0.3));
#4724=CARTESIAN_POINT('',(0.,0.41,-0.3));
#4725=CARTESIAN_POINT('',(10.,0.82,-0.3));
#4726=CARTESIAN_POINT('',(-0.1,0.82,-0.3));
#4727=CARTESIAN_POINT('',(10.,1.,-0.3));
#4728=CARTESIAN_POINT('',(10.,0.41,-0.3));
#4729=CARTESIAN_POINT('',(-0.05,1.,-0.3));
#4730=CARTESIAN_POINT('Origin',(-0.1,0.82,-0.55));
#4731=CARTESIAN_POINT('',(0.,0.82,-0.55));
#4732=CARTESIAN_POINT('',(0.,0.82,-0.275));
#4733=CARTESIAN_POINT('',(10.,0.82,-0.55));
#4734=CARTESIAN_POINT('',(-0.1,0.82,-0.55));
#4735=CARTESIAN_POINT('',(10.,0.82,-0.275));
#4736=CARTESIAN_POINT('Origin',(-0.1,0.67,-0.55));
#4737=CARTESIAN_POINT('',(0.,0.67,-0.55));
#4738=CARTESIAN_POINT('',(0.,0.335,-0.55));
#4739=CARTESIAN_POINT('',(10.,0.67,-0.55));
#4740=CARTESIAN_POINT('',(-0.1,0.67,-0.55));
#4741=CARTESIAN_POINT('',(10.,0.335,-0.55));
#4742=CARTESIAN_POINT('Origin',(-0.1,0.42,-0.3));
#4743=CARTESIAN_POINT('',(10.,0.24,-0.12));
#4744=CARTESIAN_POINT('',(0.,0.24,-0.12));
#4745=CARTESIAN_POINT('Origin',(-0.1,0.82,0.55));
#4746=CARTESIAN_POINT('',(10.,0.82,0.55));
#4747=CARTESIAN_POINT('',(-0.1,0.82,0.55));
#4748=CARTESIAN_POINT('',(10.,0.41,0.55));
#4749=CARTESIAN_POINT('Origin',(-0.1,0.82,0.3));
#4750=CARTESIAN_POINT('',(10.,0.82,0.3));
#4751=CARTESIAN_POINT('',(-0.1,0.82,0.3));
#4752=CARTESIAN_POINT('',(10.,0.82,0.15));
#4753=CARTESIAN_POINT('Origin',(-0.1,1.05,0.3));
#4754=CARTESIAN_POINT('',(10.,1.,0.3));
#4755=CARTESIAN_POINT('',(-0.05,1.,0.3));
#4756=CARTESIAN_POINT('',(10.,0.525,0.3));
#4757=CARTESIAN_POINT('Origin',(-0.1,-0.3,-0.82));
#4758=CARTESIAN_POINT('',(10.,-0.3,-0.82));
#4759=CARTESIAN_POINT('',(-0.1,-0.3,-0.82));
#4760=CARTESIAN_POINT('',(10.,-0.3,-1.));
#4761=CARTESIAN_POINT('',(10.,-0.3,-0.41));
#4762=CARTESIAN_POINT('',(-0.05,-0.3,-1.));
#4763=CARTESIAN_POINT('Origin',(-0.1,-0.55,-0.82));
#4764=CARTESIAN_POINT('',(10.,-0.55,-0.82));
#4765=CARTESIAN_POINT('',(-0.1,-0.55,-0.82));
#4766=CARTESIAN_POINT('',(10.,-0.275,-0.82));
#4767=CARTESIAN_POINT('Origin',(-0.1,-0.55,-0.67));
#4768=CARTESIAN_POINT('',(10.,-0.55,-0.67));
#4769=CARTESIAN_POINT('',(-0.1,-0.55,-0.67));
#4770=CARTESIAN_POINT('',(10.,-0.55,-0.335));
#4771=CARTESIAN_POINT('Origin',(-0.1,-0.3,-0.42));
#4772=CARTESIAN_POINT('',(10.,-0.3,-0.42));
#4773=CARTESIAN_POINT('',(-0.1,-0.3,-0.42));
#4774=CARTESIAN_POINT('',(10.,-0.12,-0.24));
#4775=CARTESIAN_POINT('Origin',(-0.1,0.3,-0.42));
#4776=CARTESIAN_POINT('',(10.,0.3,-0.42));
#4777=CARTESIAN_POINT('',(-0.1,0.3,-0.42));
#4778=CARTESIAN_POINT('',(10.,0.15,-0.42));
#4779=CARTESIAN_POINT('Origin',(-0.1,0.55,-0.67));
#4780=CARTESIAN_POINT('',(0.,0.55,-0.67));
#4781=CARTESIAN_POINT('',(0.,0.245,-0.365));
#4782=CARTESIAN_POINT('',(10.,0.55,-0.67));
#4783=CARTESIAN_POINT('',(-0.1,0.55,-0.67));
#4784=CARTESIAN_POINT('',(10.,0.245,-0.365));
#4785=CARTESIAN_POINT('Origin',(-0.1,0.55,-0.82));
#4786=CARTESIAN_POINT('',(0.,0.55,-0.82));
#4787=CARTESIAN_POINT('',(0.,0.55,-0.41));
#4788=CARTESIAN_POINT('',(10.,0.55,-0.82));
#4789=CARTESIAN_POINT('',(-0.1,0.55,-0.82));
#4790=CARTESIAN_POINT('',(10.,0.55,-0.41));
#4791=CARTESIAN_POINT('Origin',(-0.1,0.3,-0.82));
#4792=CARTESIAN_POINT('',(0.,0.3,-0.82));
#4793=CARTESIAN_POINT('',(0.,0.15,-0.82));
#4794=CARTESIAN_POINT('',(10.,0.3,-0.82));
#4795=CARTESIAN_POINT('',(-0.1,0.3,-0.82));
#4796=CARTESIAN_POINT('',(10.,0.15,-0.82));
#4797=CARTESIAN_POINT('Origin',(-0.1,0.3,-1.05));
#4798=CARTESIAN_POINT('',(0.,0.3,-1.));
#4799=CARTESIAN_POINT('',(0.,0.3,-0.525));
#4800=CARTESIAN_POINT('',(10.,0.3,-1.));
#4801=CARTESIAN_POINT('',(-0.05,0.3,-1.));
#4802=CARTESIAN_POINT('',(10.,0.3,-0.525));
#4803=CARTESIAN_POINT('Origin',(-0.1,-0.82,0.3));
#4804=CARTESIAN_POINT('',(10.,-0.82,0.3));
#4805=CARTESIAN_POINT('',(-0.1,-0.82,0.3));
#4806=CARTESIAN_POINT('',(10.,-1.,0.3));
#4807=CARTESIAN_POINT('',(10.,-0.41,0.3));
#4808=CARTESIAN_POINT('',(-0.05,-1.,0.3));
#4809=CARTESIAN_POINT('Origin',(-0.1,-0.82,0.55));
#4810=CARTESIAN_POINT('',(10.,-0.82,0.55));
#4811=CARTESIAN_POINT('',(-0.1,-0.82,0.55));
#4812=CARTESIAN_POINT('',(10.,-0.82,0.275));
#4813=CARTESIAN_POINT('Origin',(-0.1,-0.67,0.55));
#4814=CARTESIAN_POINT('',(10.,-0.67,0.55));
#4815=CARTESIAN_POINT('',(-0.1,-0.67,0.55));
#4816=CARTESIAN_POINT('',(10.,-0.335,0.55));
#4817=CARTESIAN_POINT('Origin',(-0.1,-0.42,0.3));
#4818=CARTESIAN_POINT('',(10.,-0.42,0.3));
#4819=CARTESIAN_POINT('',(-0.1,-0.42,0.3));
#4820=CARTESIAN_POINT('',(10.,-0.24,0.12));
#4821=CARTESIAN_POINT('Origin',(-0.1,-0.42,-0.3));
#4822=CARTESIAN_POINT('',(10.,-0.42,-0.3));
#4823=CARTESIAN_POINT('',(-0.1,-0.42,-0.3));
#4824=CARTESIAN_POINT('',(10.,-0.42,-0.15));
#4825=CARTESIAN_POINT('Origin',(-0.1,-0.67,-0.55));
#4826=CARTESIAN_POINT('',(10.,-0.67,-0.55));
#4827=CARTESIAN_POINT('',(-0.1,-0.67,-0.55));
#4828=CARTESIAN_POINT('',(10.,-0.365,-0.245));
#4829=CARTESIAN_POINT('Origin',(-0.1,-0.82,-0.55));
#4830=CARTESIAN_POINT('',(10.,-0.82,-0.55));
#4831=CARTESIAN_POINT('',(-0.1,-0.82,-0.55));
#4832=CARTESIAN_POINT('',(10.,-0.41,-0.55));
#4833=CARTESIAN_POINT('Origin',(-0.1,-0.82,-0.3));
#4834=CARTESIAN_POINT('',(10.,-0.82,-0.3));
#4835=CARTESIAN_POINT('',(-0.1,-0.82,-0.3));
#4836=CARTESIAN_POINT('',(10.,-0.82,-0.15));
#4837=CARTESIAN_POINT('Origin',(-0.1,-1.05,-0.3));
#4838=CARTESIAN_POINT('',(10.,-1.,-0.3));
#4839=CARTESIAN_POINT('',(-0.05,-1.,-0.3));
#4840=CARTESIAN_POINT('',(10.,-0.525,-0.3));
#4841=CARTESIAN_POINT('Origin',(-0.1,0.3,0.82));
#4842=CARTESIAN_POINT('',(10.,0.3,0.82));
#4843=CARTESIAN_POINT('',(-0.1,0.3,0.82));
#4844=CARTESIAN_POINT('',(10.,0.3,1.));
#4845=CARTESIAN_POINT('',(10.,0.3,0.41));
#4846=CARTESIAN_POINT('',(-0.05,0.3,1.));
#4847=CARTESIAN_POINT('Origin',(-0.1,0.55,0.82));
#4848=CARTESIAN_POINT('',(10.,0.55,0.82));
#4849=CARTESIAN_POINT('',(-0.1,0.55,0.82));
#4850=CARTESIAN_POINT('',(10.,0.275,0.82));
#4851=CARTESIAN_POINT('Origin',(-0.1,0.55,0.67));
#4852=CARTESIAN_POINT('',(10.,0.55,0.335));
#4853=CARTESIAN_POINT('Origin',(-0.1,-0.55,0.67));
#4854=CARTESIAN_POINT('',(10.,-0.55,0.67));
#4855=CARTESIAN_POINT('',(-0.1,-0.55,0.67));
#4856=CARTESIAN_POINT('',(10.,-0.245,0.365));
#4857=CARTESIAN_POINT('Origin',(-0.1,-0.55,0.82));
#4858=CARTESIAN_POINT('',(10.,-0.55,0.82));
#4859=CARTESIAN_POINT('',(-0.1,-0.55,0.82));
#4860=CARTESIAN_POINT('',(10.,-0.55,0.41));
#4861=CARTESIAN_POINT('Origin',(-0.1,-0.3,0.82));
#4862=CARTESIAN_POINT('',(10.,-0.3,0.82));
#4863=CARTESIAN_POINT('',(-0.1,-0.3,0.82));
#4864=CARTESIAN_POINT('',(10.,-0.15,0.82));
#4865=CARTESIAN_POINT('Origin',(-0.1,-0.3,1.05));
#4866=CARTESIAN_POINT('',(10.,-0.3,1.));
#4867=CARTESIAN_POINT('',(-0.05,-0.3,1.));
#4868=CARTESIAN_POINT('',(10.,-0.3,0.525));
#4869=CARTESIAN_POINT('Origin',(-0.1,0.,0.));
#4870=CARTESIAN_POINT('',(10.,2.57175827820944E-17,0.21));
#4871=CARTESIAN_POINT('',(-0.1,-2.57175827820944E-17,0.21));
#4872=CARTESIAN_POINT('Origin',(10.,0.,0.));
#4873=CARTESIAN_POINT('Origin',(0.,1.,-1.));
#4874=CARTESIAN_POINT('',(10.,1.,1.));
#4875=CARTESIAN_POINT('',(0.,1.,1.));
#4876=CARTESIAN_POINT('',(10.,1.,-1.));
#4877=CARTESIAN_POINT('Origin',(0.,1.,-1.));
#4878=CARTESIAN_POINT('',(10.,1.,-1.));
#4879=CARTESIAN_POINT('',(10.,1.,-1.));
#4880=CARTESIAN_POINT('',(0.,1.,-1.));
#4881=CARTESIAN_POINT('',(0.,1.,-1.));
#4882=CARTESIAN_POINT('',(0.,1.,-1.));
#4883=CARTESIAN_POINT('Origin',(0.,-1.,-1.));
#4884=CARTESIAN_POINT('',(0.,-1.,-1.));
#4885=CARTESIAN_POINT('',(10.,-1.,-1.));
#4886=CARTESIAN_POINT('Origin',(0.,-1.,-1.));
#4887=CARTESIAN_POINT('',(10.,-1.,-1.));
#4888=CARTESIAN_POINT('',(10.,-1.,-1.));
#4889=CARTESIAN_POINT('',(0.,-1.,-1.));
#4890=CARTESIAN_POINT('Origin',(0.,-1.,1.));
#4891=CARTESIAN_POINT('',(10.,-1.,1.));
#4892=CARTESIAN_POINT('Origin',(0.,-1.,1.));
#4893=CARTESIAN_POINT('',(10.,-1.,1.));
#4894=CARTESIAN_POINT('',(10.,-1.,1.));
#4895=CARTESIAN_POINT('',(0.,-1.,1.));
#4896=CARTESIAN_POINT('Origin',(0.,1.,1.));
#4897=CARTESIAN_POINT('',(10.,1.,1.));
#4898=CARTESIAN_POINT('Origin',(0.,1.,1.));
#4899=CARTESIAN_POINT('',(10.,1.,1.));
#4900=CARTESIAN_POINT('Origin',(10.,0.,0.));
#4901=CARTESIAN_POINT('Origin',(0.,0.,0.));
#5479=UNCERTAINTY_MEASURE_WITH_UNIT(LENGTH_MEASURE(0.001),#5503,
'DISTANCE_ACCURACY_VALUE',
'Maximum model space distance between geometric entities at asserted c
onnectivities');
#5489=UNCERTAINTY_MEASURE_WITH_UNIT(LENGTH_MEASURE(0.001),#5503,
'DISTANCE_ACCURACY_VALUE',
'Maximum model space distance between geometric entities at asserted c
onnectivities');
#5492=(
GEOMETRIC_REPRESENTATION_CONTEXT(3)
GLOBAL_UNCERTAINTY_ASSIGNED_CONTEXT((#5479))
GLOBAL_UNIT_ASSIGNED_CONTEXT((#5503,#5505,#5506))
REPRESENTATION_CONTEXT('','3D')
);
#5502=(
GEOMETRIC_REPRESENTATION_CONTEXT(3)
GLOBAL_UNCERTAINTY_ASSIGNED_CONTEXT((#5489))
GLOBAL_UNIT_ASSIGNED_CONTEXT((#5503,#5505,#5506))
REPRESENTATION_CONTEXT('','3D')
);
#5503=(
LENGTH_UNIT()
NAMED_UNIT(*)
SI_UNIT(.CENTI.,.METRE.)
);
#5505=(
NAMED_UNIT(*)
PLANE_ANGLE_UNIT()
SI_UNIT($,.RADIAN.)
);
#5506=(
NAMED_UNIT(*)
SI_UNIT($,.STERADIAN.)
SOLID_ANGLE_UNIT()
);
#5509=SHAPE_DEFINITION_REPRESENTATION(#5521,#5556);
#5521=PRODUCT_DEFINITION_SHAPE('',$,#5569);
#5556=SHAPE_REPRESENTATION('',(#3344),#5492);
#5566=PRODUCT_DEFINITION_CONTEXT('part definition',#5604,'design');
#5569=PRODUCT_DEFINITION('Slotted Extrusion - 20 x 20 x 100 mm',
'Slotted Extrusion - 20 x 20 x 100 mm',#5581,#5566);
#5581=PRODUCT_DEFINITION_FORMATION('',$,#5608);
#5604=APPLICATION_CONTEXT(
'Core Data for Automotive Mechanical Design Process');
#5605=PRODUCT_CONTEXT('part definition',#5604,'mechanical');
#5608=PRODUCT('Slotted Extrusion - 20 x 20 x 100 mm',
'Slotted Extrusion - 20 x 20 x 100 mm',
'Slotted Extrusion - 20 x 20 x 100 mm',(#5605));
#5702=COLOUR_RGB('Off White',0.89,0.88,0.83);
#5703=FILL_AREA_STYLE_COLOUR('',#5702);
#5704=FILL_AREA_STYLE('',(#5703));
#5705=SURFACE_STYLE_FILL_AREA(#5704);
#5706=SURFACE_SIDE_STYLE('',(#5705));
#5707=SURFACE_STYLE_USAGE(.BOTH.,#5706);
#5708=PRESENTATION_STYLE_ASSIGNMENT((#5707));
ENDSEC;
END-ISO-10303-21;
